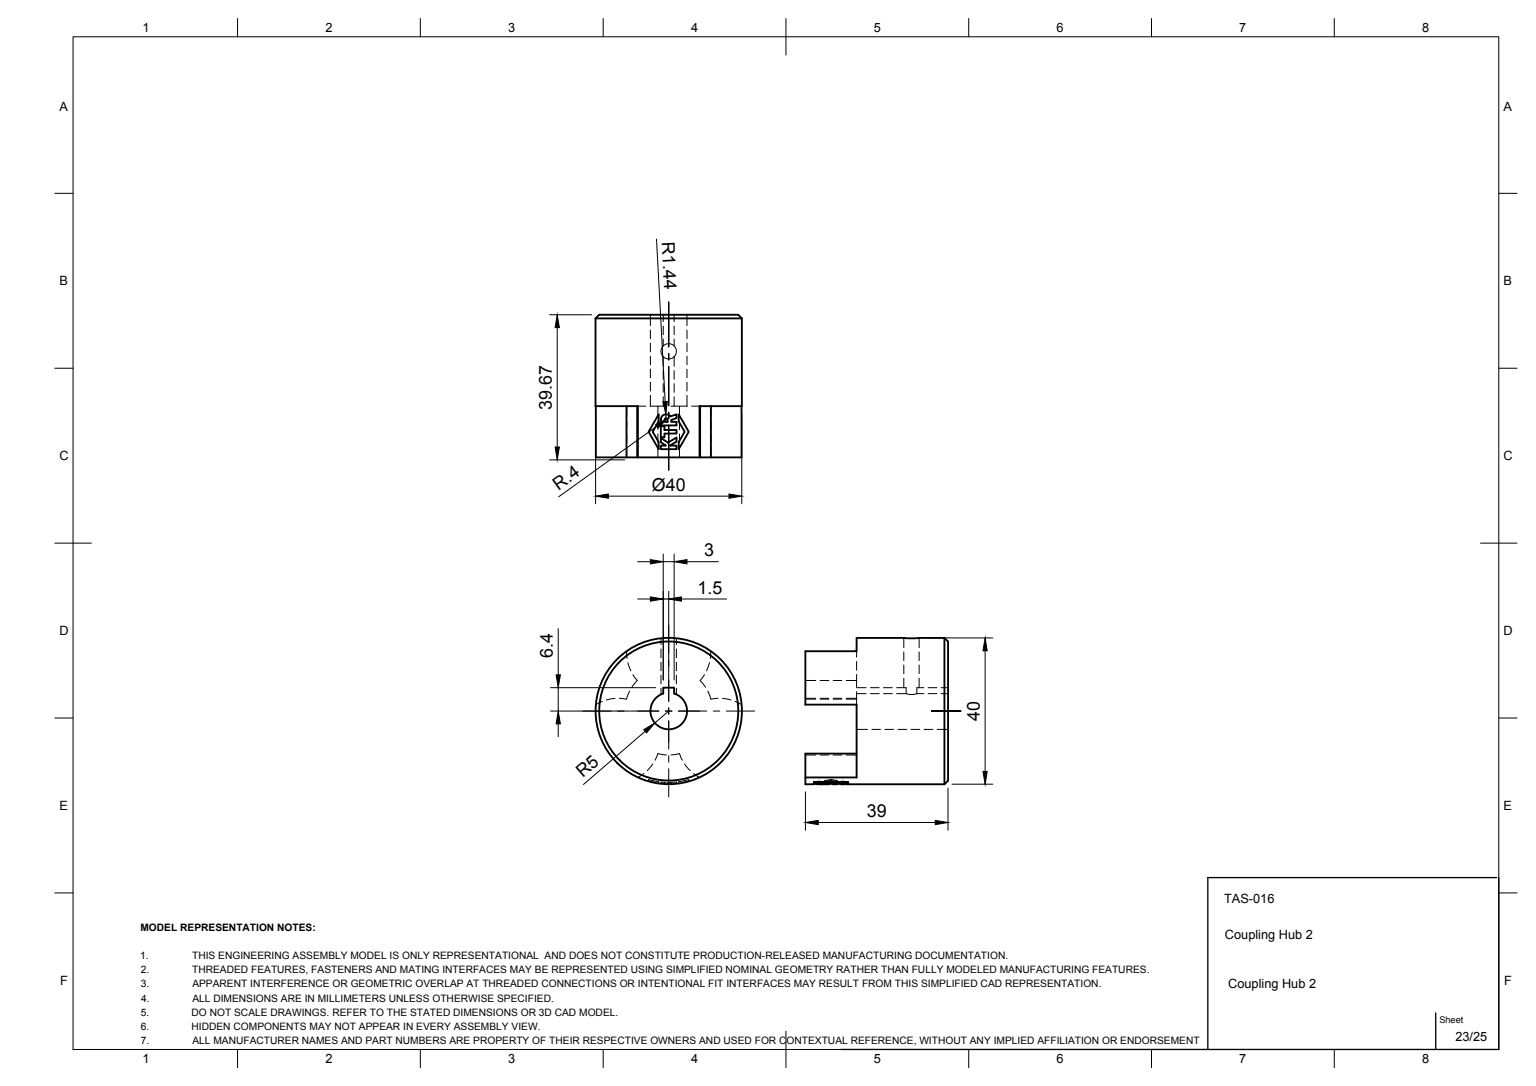
ISO-10303-21;
HEADER;
/* Generated by software containing ST-Developer
 * from STEP Tools, Inc. (www.steptools.com) 
 */

FILE_DESCRIPTION(
/* description */ ('STEP AP214'),
/* implementation_level */ '2;1');

FILE_NAME(
/* name */ 'Coupling Hub 2.step',
/* time_stamp */ '2026-11-15T14:55:55-08:00',
/* author */ (''),
/* organization */ (''),
/* preprocessor_version */ 'ST-DEVELOPER v20.2',
/* originating_system */ 'Autodesk Translation Framework v15.17.0.0',
/* authorisation */ '');

FILE_SCHEMA (('AUTOMOTIVE_DESIGN { 1 0 10303 214 3 1 1 }'));
ENDSEC;

DATA;
#10=MECHANICAL_DESIGN_GEOMETRIC_PRESENTATION_REPRESENTATION('',(#943),#57079);
#90=ELLIPSE('',#25887,40.0000000130718,20.0000000134373);
#91=ELLIPSE('',#25888,39.9999999264935,19.999999930827);
#92=ELLIPSE('',#25889,39.9999999974836,19.9999999977429);
#93=ELLIPSE('',#25890,40.0000000047116,20.0000000045204);
#94=ELLIPSE('',#25891,23.3867968076182,20.);
#95=ELLIPSE('',#25892,23.386796807644,20.);
#96=ELLIPSE('',#25896,24.1243589702644,20.);
#97=ELLIPSE('',#25897,24.124358970134,20.);
#98=ELLIPSE('',#25898,39.999999976902,19.9999999789991);
#99=ELLIPSE('',#25899,40.0000000049323,20.0000000047275);
#100=ELLIPSE('',#25900,39.9999999975502,19.999999997805);
#101=ELLIPSE('',#25901,39.9999999389236,19.9999999427079);
#102=ELLIPSE('',#25916,22.8021268874529,19.5);
#103=ELLIPSE('',#25919,22.8021268874277,19.5);
#104=ELLIPSE('',#25922,23.5212499960078,19.5);
#105=ELLIPSE('',#25932,23.5212499958807,19.5);
#106=ELLIPSE('',#25935,39.0000000024375,19.500000002367);
#107=ELLIPSE('',#25936,39.0000000667235,19.500000064201);
#108=ELLIPSE('',#25937,38.9999999995571,19.5000000004649);
#109=ELLIPSE('',#25938,38.999999996593,19.4999999968888);
#110=ELLIPSE('',#25947,38.9999999955418,19.4999999959037);
#111=ELLIPSE('',#25949,38.999999997527,19.4999999977637);
#112=ELLIPSE('',#25952,39.0000000253793,19.5000000249782);
#113=ELLIPSE('',#25954,39.0000000418424,19.5000000405918);
#851=B_SPLINE_CURVE_WITH_KNOTS('',3,(#52270,#52271,#52272,#52273,#52274,
#52275,#52276,#52277,#52278,#52279,#52280,#52281,#52282,#52283,#52284,#52285,
#52286,#52287),.UNSPECIFIED.,.F.,.F.,(4,2,2,2,2,2,2,2,4),(0.,0.0151925643701926,
0.0303851287403852,0.045584296496648,0.0607834642529108,0.0759910091953897,
0.0911985541378687,0.106391953286869,0.121585352435869),.UNSPECIFIED.);
#852=B_SPLINE_CURVE_WITH_KNOTS('',3,(#52369,#52370,#52371,#52372,#52373,
#52374,#52375,#52376,#52377,#52378,#52379),.UNSPECIFIED.,.F.,.F.,(4,2,3,
2,4),(-0.15830486583654,-0.080247501535826,0.,0.0802475015358259,0.15830486583654),
 .UNSPECIFIED.);
#853=B_SPLINE_CURVE_WITH_KNOTS('',3,(#52384,#52385,#52386,#52387,#52388,
#52389,#52390,#52391,#52392,#52393),.UNSPECIFIED.,.F.,.F.,(4,2,2,2,4),(0.483273505725753,
0.561330870026467,0.641578371562293,0.721825873098119,0.799883237398833),
 .UNSPECIFIED.);
#854=B_SPLINE_CURVE_WITH_KNOTS('',3,(#52421,#52422,#52423,#52424,#52425,
#52426,#52427,#52428,#52429,#52430,#52431,#52432,#52433,#52434,#52435,#52436,
#52437,#52438),.UNSPECIFIED.,.F.,.F.,(4,2,2,2,2,2,2,2,4),(0.316667444606564,
0.395834141831916,0.475000839057267,0.554167864135198,0.633334889213128,
0.712501914291059,0.791668939368989,0.870835636594341,0.950002333819692),
 .UNSPECIFIED.);
#855=B_SPLINE_CURVE_WITH_KNOTS('',3,(#52440,#52441,#52442,#52443,#52444,
#52445,#52446,#52447,#52448,#52449),.UNSPECIFIED.,.F.,.F.,(4,2,2,2,4),(-1.26666977842626,
-1.18750275334833,-1.10833572827039,-1.02916903104504,-0.950002333819692),
 .UNSPECIFIED.);
#856=B_SPLINE_CURVE_WITH_KNOTS('',3,(#52450,#52451,#52452,#52453,#52454,
#52455,#52456,#52457,#52458,#52459),.UNSPECIFIED.,.F.,.F.,(4,2,2,2,4),(0.950002333819692,
1.02916903104504,1.1083357282704,1.18750275334833,1.26666977842626),
 .UNSPECIFIED.);
#857=B_SPLINE_CURVE_WITH_KNOTS('',3,(#52465,#52466,#52467,#52468,#52469,
#52470,#52471,#52472,#52473,#52474,#52475,#52476,#52477,#52478,#52479,#52480),
 .UNSPECIFIED.,.F.,.F.,(4,2,2,2,2,2,2,4),(-0.779979052988675,-0.757912790448093,
-0.703814302563526,-0.64971581467896,-0.595510917659987,-0.541306020641014,
-0.487185868025911,-0.433065715410808),.UNSPECIFIED.);
#858=B_SPLINE_CURVE_WITH_KNOTS('',3,(#52703,#52704,#52705,#52706,#52707,
#52708,#52709,#52710,#52711,#52712,#52713,#52714,#52715,#52716,#52717,#52718),
 .UNSPECIFIED.,.F.,.F.,(4,2,2,2,2,2,2,4),(0.43308109743951,0.487202501340474,
0.541323905241438,0.595534461493003,0.649745017744569,0.703843614398011,
0.757942211051454,0.780009479202147),.UNSPECIFIED.);
#859=B_SPLINE_CURVE_WITH_KNOTS('',3,(#52750,#52751,#52752,#52753,#52754,
#52755,#52756,#52757,#52758,#52759,#52760,#52761,#52762,#52763,#52764,#52765,
#52766,#52767),.UNSPECIFIED.,.F.,.F.,(4,2,2,2,2,2,2,2,4),(0.121587491028333,
0.136780909575281,0.151974328122229,0.167182628159423,0.182390928196617,
0.197590414964019,0.212789901731421,0.227982441894043,0.243174982056666),
 .UNSPECIFIED.);
#883=SHAPE_REPRESENTATION_RELATIONSHIP('SRR','None',#57271,#912);
#912=ADVANCED_BREP_SHAPE_REPRESENTATION('',(#980),#57063);
#943=STYLED_ITEM('',(#57444),#980);
#980=MANIFOLD_SOLID_BREP('Body1',#24543);
#1149=FACE_BOUND('',#4239,.T.);
#1150=FACE_BOUND('',#4251,.T.);
#1151=FACE_BOUND('',#4264,.T.);
#1152=FACE_BOUND('',#4265,.T.);
#1153=FACE_BOUND('',#4266,.T.);
#1154=FACE_BOUND('',#4267,.T.);
#1155=FACE_BOUND('',#4268,.T.);
#1156=FACE_BOUND('',#4318,.T.);
#1609=PLANE('',#25821);
#1610=PLANE('',#25826);
#1611=PLANE('',#25833);
#1612=PLANE('',#25838);
#1613=PLANE('',#25855);
#1614=PLANE('',#25868);
#1615=PLANE('',#25869);
#1616=PLANE('',#25870);
#1617=PLANE('',#25872);
#1618=PLANE('',#25875);
#1619=PLANE('',#25876);
#1620=PLANE('',#25907);
#1621=PLANE('',#25908);
#1622=PLANE('',#25909);
#1623=PLANE('',#25910);
#1624=PLANE('',#25911);
#1625=PLANE('',#25912);
#1626=PLANE('',#25913);
#1627=PLANE('',#25914);
#1628=PLANE('',#25915);
#1629=PLANE('',#25917);
#1630=PLANE('',#25918);
#1631=PLANE('',#25920);
#1632=PLANE('',#25921);
#1633=PLANE('',#25923);
#1634=PLANE('',#25925);
#1635=PLANE('',#25926);
#1636=PLANE('',#25928);
#1637=PLANE('',#25929);
#1638=PLANE('',#25931);
#1639=PLANE('',#25939);
#1640=PLANE('',#25940);
#1641=PLANE('',#25941);
#1642=PLANE('',#25942);
#1643=PLANE('',#25943);
#1644=PLANE('',#25944);
#1645=PLANE('',#25945);
#1646=PLANE('',#25946);
#1647=PLANE('',#25948);
#1648=PLANE('',#25950);
#1649=PLANE('',#25951);
#1650=PLANE('',#25953);
#1651=PLANE('',#25956);
#1652=PLANE('',#25958);
#1653=PLANE('',#25959);
#1654=PLANE('',#25962);
#1655=PLANE('',#25963);
#1656=PLANE('',#25965);
#1657=PLANE('',#25966);
#1658=PLANE('',#25968);
#1659=PLANE('',#25969);
#1660=PLANE('',#25971);
#1661=PLANE('',#25973);
#2123=CONICAL_SURFACE('',#25829,19.5,0.785398163397448);
#2713=FACE_OUTER_BOUND('',#4237,.T.);
#2714=FACE_OUTER_BOUND('',#4238,.T.);
#2715=FACE_OUTER_BOUND('',#4240,.T.);
#2716=FACE_OUTER_BOUND('',#4241,.T.);
#2717=FACE_OUTER_BOUND('',#4242,.T.);
#2718=FACE_OUTER_BOUND('',#4243,.T.);
#2719=FACE_OUTER_BOUND('',#4244,.T.);
#2720=FACE_OUTER_BOUND('',#4245,.T.);
#2721=FACE_OUTER_BOUND('',#4246,.T.);
#2722=FACE_OUTER_BOUND('',#4247,.T.);
#2723=FACE_OUTER_BOUND('',#4248,.T.);
#2724=FACE_OUTER_BOUND('',#4249,.T.);
#2725=FACE_OUTER_BOUND('',#4250,.T.);
#2726=FACE_OUTER_BOUND('',#4252,.T.);
#2727=FACE_OUTER_BOUND('',#4253,.T.);
#2728=FACE_OUTER_BOUND('',#4254,.T.);
#2729=FACE_OUTER_BOUND('',#4255,.T.);
#2730=FACE_OUTER_BOUND('',#4256,.T.);
#2731=FACE_OUTER_BOUND('',#4257,.T.);
#2732=FACE_OUTER_BOUND('',#4258,.T.);
#2733=FACE_OUTER_BOUND('',#4259,.T.);
#2734=FACE_OUTER_BOUND('',#4260,.T.);
#2735=FACE_OUTER_BOUND('',#4261,.T.);
#2736=FACE_OUTER_BOUND('',#4262,.T.);
#2737=FACE_OUTER_BOUND('',#4263,.T.);
#2738=FACE_OUTER_BOUND('',#4269,.T.);
#2739=FACE_OUTER_BOUND('',#4270,.T.);
#2740=FACE_OUTER_BOUND('',#4271,.T.);
#2741=FACE_OUTER_BOUND('',#4272,.T.);
#2742=FACE_OUTER_BOUND('',#4273,.T.);
#2743=FACE_OUTER_BOUND('',#4274,.T.);
#2744=FACE_OUTER_BOUND('',#4275,.T.);
#2745=FACE_OUTER_BOUND('',#4276,.T.);
#2746=FACE_OUTER_BOUND('',#4277,.T.);
#2747=FACE_OUTER_BOUND('',#4278,.T.);
#2748=FACE_OUTER_BOUND('',#4279,.T.);
#2749=FACE_OUTER_BOUND('',#4280,.T.);
#2750=FACE_OUTER_BOUND('',#4281,.T.);
#2751=FACE_OUTER_BOUND('',#4282,.T.);
#2752=FACE_OUTER_BOUND('',#4283,.T.);
#2753=FACE_OUTER_BOUND('',#4284,.T.);
#2754=FACE_OUTER_BOUND('',#4285,.T.);
#2755=FACE_OUTER_BOUND('',#4286,.T.);
#2756=FACE_OUTER_BOUND('',#4287,.T.);
#2757=FACE_OUTER_BOUND('',#4288,.T.);
#2758=FACE_OUTER_BOUND('',#4289,.T.);
#2759=FACE_OUTER_BOUND('',#4290,.T.);
#2760=FACE_OUTER_BOUND('',#4291,.T.);
#2761=FACE_OUTER_BOUND('',#4292,.T.);
#2762=FACE_OUTER_BOUND('',#4293,.T.);
#2763=FACE_OUTER_BOUND('',#4294,.T.);
#2764=FACE_OUTER_BOUND('',#4295,.T.);
#2765=FACE_OUTER_BOUND('',#4296,.T.);
#2766=FACE_OUTER_BOUND('',#4297,.T.);
#2767=FACE_OUTER_BOUND('',#4298,.T.);
#2768=FACE_OUTER_BOUND('',#4299,.T.);
#2769=FACE_OUTER_BOUND('',#4300,.T.);
#2770=FACE_OUTER_BOUND('',#4301,.T.);
#2771=FACE_OUTER_BOUND('',#4302,.T.);
#2772=FACE_OUTER_BOUND('',#4303,.T.);
#2773=FACE_OUTER_BOUND('',#4304,.T.);
#2774=FACE_OUTER_BOUND('',#4305,.T.);
#2775=FACE_OUTER_BOUND('',#4306,.T.);
#2776=FACE_OUTER_BOUND('',#4307,.T.);
#2777=FACE_OUTER_BOUND('',#4308,.T.);
#2778=FACE_OUTER_BOUND('',#4309,.T.);
#2779=FACE_OUTER_BOUND('',#4310,.T.);
#2780=FACE_OUTER_BOUND('',#4311,.T.);
#2781=FACE_OUTER_BOUND('',#4312,.T.);
#2782=FACE_OUTER_BOUND('',#4313,.T.);
#2783=FACE_OUTER_BOUND('',#4314,.T.);
#2784=FACE_OUTER_BOUND('',#4315,.T.);
#2785=FACE_OUTER_BOUND('',#4316,.T.);
#2786=FACE_OUTER_BOUND('',#4317,.T.);
#4237=EDGE_LOOP('',(#18468,#18469,#18470,#18471));
#4238=EDGE_LOOP('',(#18472));
#4239=EDGE_LOOP('',(#18473,#18474,#18475,#18476));
#4240=EDGE_LOOP('',(#18477,#18478,#18479,#18480));
#4241=EDGE_LOOP('',(#18481,#18482,#18483,#18484));
#4242=EDGE_LOOP('',(#18485,#18486,#18487,#18488));
#4243=EDGE_LOOP('',(#18489,#18490,#18491,#18492));
#4244=EDGE_LOOP('',(#18493,#18494,#18495,#18496));
#4245=EDGE_LOOP('',(#18497,#18498,#18499,#18500));
#4246=EDGE_LOOP('',(#18501,#18502,#18503,#18504));
#4247=EDGE_LOOP('',(#18505,#18506,#18507,#18508));
#4248=EDGE_LOOP('',(#18509,#18510,#18511,#18512));
#4249=EDGE_LOOP('',(#18513,#18514,#18515,#18516));
#4250=EDGE_LOOP('',(#18517,#18518,#18519,#18520,#18521,#18522,#18523,#18524,
#18525,#18526,#18527,#18528,#18529));
#4251=EDGE_LOOP('',(#18530,#18531,#18532,#18533));
#4252=EDGE_LOOP('',(#18534,#18535,#18536,#18537));
#4253=EDGE_LOOP('',(#18538,#18539,#18540,#18541));
#4254=EDGE_LOOP('',(#18542,#18543,#18544,#18545));
#4255=EDGE_LOOP('',(#18546,#18547,#18548,#18549,#18550,#18551,#18552,#18553));
#4256=EDGE_LOOP('',(#18554,#18555,#18556,#18557));
#4257=EDGE_LOOP('',(#18558,#18559,#18560,#18561));
#4258=EDGE_LOOP('',(#18562,#18563,#18564,#18565));
#4259=EDGE_LOOP('',(#18566,#18567,#18568,#18569,#18570));
#4260=EDGE_LOOP('',(#18571,#18572,#18573,#18574));
#4261=EDGE_LOOP('',(#18575,#18576,#18577,#18578));
#4262=EDGE_LOOP('',(#18579,#18580,#18581,#18582,#18583,#18584,#18585,#18586,
#18587,#18588,#18589,#18590,#18591,#18592));
#4263=EDGE_LOOP('',(#18593,#18594,#18595,#18596,#18597,#18598,#18599,#18600,
#18601,#18602,#18603,#18604,#18605,#18606,#18607,#18608,#18609,#18610,#18611,
#18612,#18613));
#4264=EDGE_LOOP('',(#18614,#18615,#18616,#18617,#18618,#18619,#18620,#18621,
#18622));
#4265=EDGE_LOOP('',(#18623,#18624,#18625,#18626,#18627,#18628,#18629,#18630));
#4266=EDGE_LOOP('',(#18631,#18632,#18633,#18634,#18635,#18636));
#4267=EDGE_LOOP('',(#18637,#18638,#18639,#18640,#18641,#18642,#18643,#18644,
#18645,#18646,#18647));
#4268=EDGE_LOOP('',(#18648,#18649,#18650,#18651,#18652,#18653));
#4269=EDGE_LOOP('',(#18654,#18655,#18656,#18657,#18658,#18659,#18660,#18661));
#4270=EDGE_LOOP('',(#18662,#18663,#18664,#18665));
#4271=EDGE_LOOP('',(#18666,#18667,#18668,#18669));
#4272=EDGE_LOOP('',(#18670,#18671,#18672,#18673));
#4273=EDGE_LOOP('',(#18674,#18675,#18676,#18677));
#4274=EDGE_LOOP('',(#18678,#18679,#18680,#18681));
#4275=EDGE_LOOP('',(#18682,#18683,#18684,#18685));
#4276=EDGE_LOOP('',(#18686,#18687,#18688,#18689));
#4277=EDGE_LOOP('',(#18690,#18691,#18692,#18693));
#4278=EDGE_LOOP('',(#18694,#18695,#18696,#18697));
#4279=EDGE_LOOP('',(#18698,#18699,#18700,#18701));
#4280=EDGE_LOOP('',(#18702,#18703,#18704,#18705));
#4281=EDGE_LOOP('',(#18706,#18707,#18708,#18709));
#4282=EDGE_LOOP('',(#18710,#18711,#18712,#18713));
#4283=EDGE_LOOP('',(#18714,#18715,#18716,#18717));
#4284=EDGE_LOOP('',(#18718,#18719,#18720,#18721));
#4285=EDGE_LOOP('',(#18722,#18723,#18724,#18725));
#4286=EDGE_LOOP('',(#18726,#18727,#18728,#18729));
#4287=EDGE_LOOP('',(#18730,#18731,#18732,#18733));
#4288=EDGE_LOOP('',(#18734,#18735,#18736,#18737));
#4289=EDGE_LOOP('',(#18738,#18739,#18740,#18741,#18742,#18743,#18744,#18745,
#18746,#18747,#18748));
#4290=EDGE_LOOP('',(#18749,#18750,#18751,#18752,#18753,#18754));
#4291=EDGE_LOOP('',(#18755,#18756,#18757,#18758));
#4292=EDGE_LOOP('',(#18759,#18760,#18761,#18762));
#4293=EDGE_LOOP('',(#18763,#18764,#18765,#18766));
#4294=EDGE_LOOP('',(#18767,#18768,#18769,#18770));
#4295=EDGE_LOOP('',(#18771,#18772,#18773,#18774));
#4296=EDGE_LOOP('',(#18775,#18776,#18777,#18778));
#4297=EDGE_LOOP('',(#18779,#18780,#18781,#18782));
#4298=EDGE_LOOP('',(#18783,#18784,#18785,#18786));
#4299=EDGE_LOOP('',(#18787,#18788,#18789,#18790));
#4300=EDGE_LOOP('',(#18791,#18792,#18793,#18794));
#4301=EDGE_LOOP('',(#18795,#18796,#18797,#18798));
#4302=EDGE_LOOP('',(#18799,#18800,#18801,#18802));
#4303=EDGE_LOOP('',(#18803,#18804,#18805,#18806,#18807,#18808));
#4304=EDGE_LOOP('',(#18809,#18810,#18811,#18812));
#4305=EDGE_LOOP('',(#18813,#18814,#18815,#18816));
#4306=EDGE_LOOP('',(#18817,#18818,#18819,#18820));
#4307=EDGE_LOOP('',(#18821,#18822,#18823,#18824));
#4308=EDGE_LOOP('',(#18825,#18826,#18827,#18828));
#4309=EDGE_LOOP('',(#18829,#18830,#18831,#18832));
#4310=EDGE_LOOP('',(#18833,#18834,#18835,#18836));
#4311=EDGE_LOOP('',(#18837,#18838,#18839,#18840));
#4312=EDGE_LOOP('',(#18841,#18842,#18843,#18844));
#4313=EDGE_LOOP('',(#18845,#18846,#18847,#18848));
#4314=EDGE_LOOP('',(#18849,#18850,#18851,#18852));
#4315=EDGE_LOOP('',(#18853,#18854,#18855,#18856));
#4316=EDGE_LOOP('',(#18857,#18858,#18859,#18860));
#4317=EDGE_LOOP('',(#18861,#18862,#18863,#18864,#18865,#18866,#18867,#18868,
#18869));
#4318=EDGE_LOOP('',(#18870,#18871,#18872,#18873));
#5864=LINE('',#52255,#7831);
#5865=LINE('',#52257,#7832);
#5866=LINE('',#52259,#7833);
#5867=LINE('',#52264,#7834);
#5868=LINE('',#52268,#7835);
#5869=LINE('',#52289,#7836);
#5870=LINE('',#52313,#7837);
#5871=LINE('',#52314,#7838);
#5872=LINE('',#52317,#7839);
#5873=LINE('',#52320,#7840);
#5874=LINE('',#52323,#7841);
#5875=LINE('',#52326,#7842);
#5876=LINE('',#52329,#7843);
#5877=LINE('',#52333,#7844);
#5878=LINE('',#52338,#7845);
#5879=LINE('',#52353,#7846);
#5880=LINE('',#52357,#7847);
#5881=LINE('',#52358,#7848);
#5882=LINE('',#52360,#7849);
#5883=LINE('',#52362,#7850);
#5884=LINE('',#52364,#7851);
#5885=LINE('',#52367,#7852);
#5886=LINE('',#52380,#7853);
#5887=LINE('',#52382,#7854);
#5888=LINE('',#52394,#7855);
#5889=LINE('',#52397,#7856);
#5890=LINE('',#52398,#7857);
#5891=LINE('',#52401,#7858);
#5892=LINE('',#52402,#7859);
#5893=LINE('',#52406,#7860);
#5894=LINE('',#52411,#7861);
#5895=LINE('',#52414,#7862);
#5896=LINE('',#52416,#7863);
#5897=LINE('',#52419,#7864);
#5898=LINE('',#52461,#7865);
#5899=LINE('',#52462,#7866);
#5900=LINE('',#52484,#7867);
#5901=LINE('',#52488,#7868);
#5902=LINE('',#52492,#7869);
#5903=LINE('',#52495,#7870);
#5904=LINE('',#52500,#7871);
#5905=LINE('',#52504,#7872);
#5906=LINE('',#52508,#7873);
#5907=LINE('',#52511,#7874);
#5908=LINE('',#52514,#7875);
#5909=LINE('',#52520,#7876);
#5910=LINE('',#52528,#7877);
#5911=LINE('',#52534,#7878);
#5912=LINE('',#52538,#7879);
#5913=LINE('',#52544,#7880);
#5914=LINE('',#52550,#7881);
#5915=LINE('',#52556,#7882);
#5916=LINE('',#52563,#7883);
#5917=LINE('',#52567,#7884);
#5918=LINE('',#52571,#7885);
#5919=LINE('',#52574,#7886);
#5920=LINE('',#52576,#7887);
#5921=LINE('',#52577,#7888);
#5922=LINE('',#52579,#7889);
#5923=LINE('',#52581,#7890);
#5924=LINE('',#52583,#7891);
#5925=LINE('',#52585,#7892);
#5926=LINE('',#52587,#7893);
#5927=LINE('',#52589,#7894);
#5928=LINE('',#52593,#7895);
#5929=LINE('',#52596,#7896);
#5930=LINE('',#52599,#7897);
#5931=LINE('',#52600,#7898);
#5932=LINE('',#52603,#7899);
#5933=LINE('',#52607,#7900);
#5934=LINE('',#52609,#7901);
#5935=LINE('',#52610,#7902);
#5936=LINE('',#52613,#7903);
#5937=LINE('',#52617,#7904);
#5938=LINE('',#52621,#7905);
#5939=LINE('',#52622,#7906);
#5940=LINE('',#52625,#7907);
#5941=LINE('',#52629,#7908);
#5942=LINE('',#52630,#7909);
#5943=LINE('',#52641,#7910);
#5944=LINE('',#52647,#7911);
#5945=LINE('',#52650,#7912);
#5946=LINE('',#52651,#7913);
#5947=LINE('',#52653,#7914);
#5948=LINE('',#52655,#7915);
#5949=LINE('',#52657,#7916);
#5950=LINE('',#52659,#7917);
#5951=LINE('',#52663,#7918);
#5952=LINE('',#52665,#7919);
#5953=LINE('',#52666,#7920);
#5954=LINE('',#52669,#7921);
#5955=LINE('',#52673,#7922);
#5956=LINE('',#52677,#7923);
#5957=LINE('',#52678,#7924);
#5958=LINE('',#52682,#7925);
#5959=LINE('',#52688,#7926);
#5960=LINE('',#52691,#7927);
#5961=LINE('',#52694,#7928);
#5962=LINE('',#52695,#7929);
#5963=LINE('',#52698,#7930);
#5964=LINE('',#52702,#7931);
#5965=LINE('',#52721,#7932);
#5966=LINE('',#52722,#7933);
#5967=LINE('',#52725,#7934);
#5968=LINE('',#52728,#7935);
#5969=LINE('',#52731,#7936);
#5970=LINE('',#52732,#7937);
#5971=LINE('',#52735,#7938);
#5972=LINE('',#52739,#7939);
#5973=LINE('',#52740,#7940);
#5974=LINE('',#52743,#7941);
#5975=LINE('',#52746,#7942);
#5976=LINE('',#52749,#7943);
#5977=LINE('',#52769,#7944);
#7831=VECTOR('',#29980,1000.);
#7832=VECTOR('',#29981,1000.);
#7833=VECTOR('',#29982,1000.);
#7834=VECTOR('',#29989,19.5);
#7835=VECTOR('',#29992,1000.);
#7836=VECTOR('',#29993,1000.);
#7837=VECTOR('',#30020,1000.);
#7838=VECTOR('',#30021,1000.);
#7839=VECTOR('',#30024,1000.);
#7840=VECTOR('',#30027,1000.);
#7841=VECTOR('',#30030,1000.);
#7842=VECTOR('',#30033,1000.);
#7843=VECTOR('',#30036,1000.);
#7844=VECTOR('',#30041,1000.);
#7845=VECTOR('',#30048,1000.);
#7846=VECTOR('',#30065,1000.);
#7847=VECTOR('',#30068,1000.);
#7848=VECTOR('',#30069,1000.);
#7849=VECTOR('',#30072,1000.);
#7850=VECTOR('',#30075,1000.);
#7851=VECTOR('',#30078,1000.);
#7852=VECTOR('',#30081,1000.);
#7853=VECTOR('',#30082,1000.);
#7854=VECTOR('',#30083,1000.);
#7855=VECTOR('',#30084,1000.);
#7856=VECTOR('',#30087,1000.);
#7857=VECTOR('',#30088,1000.);
#7858=VECTOR('',#30091,1000.);
#7859=VECTOR('',#30092,1000.);
#7860=VECTOR('',#30097,1000.);
#7861=VECTOR('',#30102,1000.);
#7862=VECTOR('',#30107,1000.);
#7863=VECTOR('',#30110,1000.);
#7864=VECTOR('',#30113,2.1);
#7865=VECTOR('',#30116,20.);
#7866=VECTOR('',#30117,20.);
#7867=VECTOR('',#30120,1000.);
#7868=VECTOR('',#30123,1000.);
#7869=VECTOR('',#30126,1000.);
#7870=VECTOR('',#30129,1000.);
#7871=VECTOR('',#30132,1000.);
#7872=VECTOR('',#30135,1000.);
#7873=VECTOR('',#30138,1000.);
#7874=VECTOR('',#30141,1000.);
#7875=VECTOR('',#30142,1000.);
#7876=VECTOR('',#30147,1000.);
#7877=VECTOR('',#30154,1000.);
#7878=VECTOR('',#30159,1000.);
#7879=VECTOR('',#30162,1000.);
#7880=VECTOR('',#30167,1000.);
#7881=VECTOR('',#30172,1000.);
#7882=VECTOR('',#30177,1000.);
#7883=VECTOR('',#30184,1000.);
#7884=VECTOR('',#30187,1000.);
#7885=VECTOR('',#30190,1000.);
#7886=VECTOR('',#30193,1000.);
#7887=VECTOR('',#30196,1000.);
#7888=VECTOR('',#30197,1000.);
#7889=VECTOR('',#30200,1000.);
#7890=VECTOR('',#30203,1000.);
#7891=VECTOR('',#30206,1000.);
#7892=VECTOR('',#30209,1000.);
#7893=VECTOR('',#30212,1000.);
#7894=VECTOR('',#30215,1000.);
#7895=VECTOR('',#30220,1000.);
#7896=VECTOR('',#30223,1000.);
#7897=VECTOR('',#30226,1000.);
#7898=VECTOR('',#30227,1000.);
#7899=VECTOR('',#30230,1000.);
#7900=VECTOR('',#30235,1000.);
#7901=VECTOR('',#30236,1000.);
#7902=VECTOR('',#30237,1000.);
#7903=VECTOR('',#30240,1000.);
#7904=VECTOR('',#30245,1000.);
#7905=VECTOR('',#30250,1000.);
#7906=VECTOR('',#30251,1000.);
#7907=VECTOR('',#30254,1000.);
#7908=VECTOR('',#30259,1000.);
#7909=VECTOR('',#30260,1000.);
#7910=VECTOR('',#30275,1000.);
#7911=VECTOR('',#30280,1000.);
#7912=VECTOR('',#30285,1000.);
#7913=VECTOR('',#30286,1000.);
#7914=VECTOR('',#30289,1000.);
#7915=VECTOR('',#30292,1000.);
#7916=VECTOR('',#30295,1000.);
#7917=VECTOR('',#30298,1000.);
#7918=VECTOR('',#30303,1000.);
#7919=VECTOR('',#30304,1000.);
#7920=VECTOR('',#30305,1000.);
#7921=VECTOR('',#30308,1000.);
#7922=VECTOR('',#30313,1000.);
#7923=VECTOR('',#30318,1000.);
#7924=VECTOR('',#30319,1000.);
#7925=VECTOR('',#30324,1000.);
#7926=VECTOR('',#30333,1000.);
#7927=VECTOR('',#30336,1000.);
#7928=VECTOR('',#30339,1000.);
#7929=VECTOR('',#30340,1000.);
#7930=VECTOR('',#30343,1000.);
#7931=VECTOR('',#30348,1000.);
#7932=VECTOR('',#30351,1000.);
#7933=VECTOR('',#30352,1000.);
#7934=VECTOR('',#30355,1000.);
#7935=VECTOR('',#30358,1000.);
#7936=VECTOR('',#30361,1000.);
#7937=VECTOR('',#30362,1000.);
#7938=VECTOR('',#30365,1000.);
#7939=VECTOR('',#30370,1000.);
#7940=VECTOR('',#30371,1000.);
#7941=VECTOR('',#30374,1000.);
#7942=VECTOR('',#30379,1000.);
#7943=VECTOR('',#30382,1000.);
#7944=VECTOR('',#30385,1000.);
#9610=CIRCLE('',#25822,11.5);
#9611=CIRCLE('',#25823,20.);
#9612=CIRCLE('',#25824,11.5);
#9613=CIRCLE('',#25825,12.);
#9614=CIRCLE('',#25827,19.);
#9615=CIRCLE('',#25828,5.);
#9616=CIRCLE('',#25830,20.);
#9617=CIRCLE('',#25832,20.);
#9618=CIRCLE('',#25834,11.5);
#9619=CIRCLE('',#25835,20.);
#9620=CIRCLE('',#25836,11.5);
#9621=CIRCLE('',#25837,12.);
#9622=CIRCLE('',#25839,11.5);
#9623=CIRCLE('',#25840,12.);
#9624=CIRCLE('',#25841,11.5);
#9625=CIRCLE('',#25842,20.);
#9626=CIRCLE('',#25844,11.5);
#9627=CIRCLE('',#25846,12.);
#9628=CIRCLE('',#25848,12.);
#9629=CIRCLE('',#25850,12.);
#9630=CIRCLE('',#25852,11.5);
#9631=CIRCLE('',#25854,11.5);
#9632=CIRCLE('',#25856,20.);
#9633=CIRCLE('',#25857,11.5);
#9634=CIRCLE('',#25858,20.);
#9635=CIRCLE('',#25859,20.);
#9636=CIRCLE('',#25860,11.5);
#9637=CIRCLE('',#25861,20.);
#9638=CIRCLE('',#25862,11.5);
#9639=CIRCLE('',#25863,5.);
#9640=CIRCLE('',#25871,2.1);
#9641=CIRCLE('',#25873,2.1);
#9642=CIRCLE('',#25874,2.1);
#9643=CIRCLE('',#25879,22.3311974134124);
#9644=CIRCLE('',#25880,22.32884051476);
#9645=CIRCLE('',#25881,20.);
#9646=CIRCLE('',#25882,20.);
#9647=CIRCLE('',#25883,20.);
#9648=CIRCLE('',#25884,20.);
#9649=CIRCLE('',#25885,20.);
#9650=CIRCLE('',#25886,20.);
#9651=CIRCLE('',#25893,20.);
#9652=CIRCLE('',#25894,20.);
#9653=CIRCLE('',#25895,20.);
#9654=CIRCLE('',#25903,19.5);
#9655=CIRCLE('',#25904,19.5);
#9656=CIRCLE('',#25905,19.5);
#9657=CIRCLE('',#25906,19.5);
#9658=CIRCLE('',#25924,19.5);
#9659=CIRCLE('',#25927,19.5);
#9660=CIRCLE('',#25930,19.5);
#9661=CIRCLE('',#25957,21.7696935948967);
#9662=CIRCLE('',#25960,21.7721107487055);
#9663=CIRCLE('',#25964,19.5);
#9664=CIRCLE('',#25967,19.5);
#9665=CIRCLE('',#25970,19.5);
#11088=VERTEX_POINT('',#52242);
#11089=VERTEX_POINT('',#52243);
#11090=VERTEX_POINT('',#52245);
#11091=VERTEX_POINT('',#52247);
#11092=VERTEX_POINT('',#52251);
#11093=VERTEX_POINT('',#52253);
#11094=VERTEX_POINT('',#52254);
#11095=VERTEX_POINT('',#52256);
#11096=VERTEX_POINT('',#52258);
#11097=VERTEX_POINT('',#52262);
#11098=VERTEX_POINT('',#52266);
#11099=VERTEX_POINT('',#52267);
#11100=VERTEX_POINT('',#52269);
#11101=VERTEX_POINT('',#52288);
#11102=VERTEX_POINT('',#52292);
#11103=VERTEX_POINT('',#52293);
#11104=VERTEX_POINT('',#52295);
#11105=VERTEX_POINT('',#52297);
#11106=VERTEX_POINT('',#52301);
#11107=VERTEX_POINT('',#52302);
#11108=VERTEX_POINT('',#52304);
#11109=VERTEX_POINT('',#52306);
#11110=VERTEX_POINT('',#52310);
#11111=VERTEX_POINT('',#52311);
#11112=VERTEX_POINT('',#52316);
#11113=VERTEX_POINT('',#52318);
#11114=VERTEX_POINT('',#52322);
#11115=VERTEX_POINT('',#52324);
#11116=VERTEX_POINT('',#52328);
#11117=VERTEX_POINT('',#52332);
#11118=VERTEX_POINT('',#52336);
#11119=VERTEX_POINT('',#52340);
#11120=VERTEX_POINT('',#52342);
#11121=VERTEX_POINT('',#52344);
#11122=VERTEX_POINT('',#52346);
#11123=VERTEX_POINT('',#52351);
#11124=VERTEX_POINT('',#52352);
#11125=VERTEX_POINT('',#52354);
#11126=VERTEX_POINT('',#52356);
#11127=VERTEX_POINT('',#52366);
#11128=VERTEX_POINT('',#52368);
#11129=VERTEX_POINT('',#52381);
#11130=VERTEX_POINT('',#52383);
#11131=VERTEX_POINT('',#52396);
#11132=VERTEX_POINT('',#52400);
#11133=VERTEX_POINT('',#52404);
#11134=VERTEX_POINT('',#52408);
#11135=VERTEX_POINT('',#52410);
#11136=VERTEX_POINT('',#52418);
#11137=VERTEX_POINT('',#52420);
#11138=VERTEX_POINT('',#52439);
#11139=VERTEX_POINT('',#52463);
#11140=VERTEX_POINT('',#52464);
#11141=VERTEX_POINT('',#52481);
#11142=VERTEX_POINT('',#52483);
#11143=VERTEX_POINT('',#52485);
#11144=VERTEX_POINT('',#52487);
#11145=VERTEX_POINT('',#52489);
#11146=VERTEX_POINT('',#52491);
#11147=VERTEX_POINT('',#52493);
#11148=VERTEX_POINT('',#52496);
#11149=VERTEX_POINT('',#52497);
#11150=VERTEX_POINT('',#52499);
#11151=VERTEX_POINT('',#52501);
#11152=VERTEX_POINT('',#52503);
#11153=VERTEX_POINT('',#52505);
#11154=VERTEX_POINT('',#52507);
#11155=VERTEX_POINT('',#52509);
#11156=VERTEX_POINT('',#52512);
#11157=VERTEX_POINT('',#52513);
#11158=VERTEX_POINT('',#52515);
#11159=VERTEX_POINT('',#52517);
#11160=VERTEX_POINT('',#52519);
#11161=VERTEX_POINT('',#52521);
#11162=VERTEX_POINT('',#52524);
#11163=VERTEX_POINT('',#52525);
#11164=VERTEX_POINT('',#52527);
#11165=VERTEX_POINT('',#52529);
#11166=VERTEX_POINT('',#52531);
#11167=VERTEX_POINT('',#52533);
#11168=VERTEX_POINT('',#52535);
#11169=VERTEX_POINT('',#52537);
#11170=VERTEX_POINT('',#52539);
#11171=VERTEX_POINT('',#52541);
#11172=VERTEX_POINT('',#52543);
#11173=VERTEX_POINT('',#52546);
#11174=VERTEX_POINT('',#52547);
#11175=VERTEX_POINT('',#52549);
#11176=VERTEX_POINT('',#52551);
#11177=VERTEX_POINT('',#52553);
#11178=VERTEX_POINT('',#52555);
#11179=VERTEX_POINT('',#52559);
#11180=VERTEX_POINT('',#52560);
#11181=VERTEX_POINT('',#52562);
#11182=VERTEX_POINT('',#52564);
#11183=VERTEX_POINT('',#52566);
#11184=VERTEX_POINT('',#52568);
#11185=VERTEX_POINT('',#52570);
#11186=VERTEX_POINT('',#52572);
#11187=VERTEX_POINT('',#52592);
#11188=VERTEX_POINT('',#52594);
#11189=VERTEX_POINT('',#52598);
#11190=VERTEX_POINT('',#52602);
#11191=VERTEX_POINT('',#52606);
#11192=VERTEX_POINT('',#52608);
#11193=VERTEX_POINT('',#52612);
#11194=VERTEX_POINT('',#52616);
#11195=VERTEX_POINT('',#52620);
#11196=VERTEX_POINT('',#52624);
#11197=VERTEX_POINT('',#52628);
#11198=VERTEX_POINT('',#52637);
#11199=VERTEX_POINT('',#52638);
#11200=VERTEX_POINT('',#52640);
#11201=VERTEX_POINT('',#52642);
#11202=VERTEX_POINT('',#52644);
#11203=VERTEX_POINT('',#52646);
#11204=VERTEX_POINT('',#52662);
#11205=VERTEX_POINT('',#52664);
#11206=VERTEX_POINT('',#52668);
#11207=VERTEX_POINT('',#52672);
#11208=VERTEX_POINT('',#52676);
#11209=VERTEX_POINT('',#52680);
#11210=VERTEX_POINT('',#52687);
#11211=VERTEX_POINT('',#52689);
#11212=VERTEX_POINT('',#52693);
#11213=VERTEX_POINT('',#52697);
#11214=VERTEX_POINT('',#52701);
#11215=VERTEX_POINT('',#52720);
#11216=VERTEX_POINT('',#52724);
#11217=VERTEX_POINT('',#52726);
#11218=VERTEX_POINT('',#52730);
#11219=VERTEX_POINT('',#52734);
#11220=VERTEX_POINT('',#52738);
#11221=VERTEX_POINT('',#52742);
#11222=VERTEX_POINT('',#52748);
#13779=EDGE_CURVE('',#11088,#11089,#9610,.T.);
#13780=EDGE_CURVE('',#11090,#11089,#9611,.T.);
#13781=EDGE_CURVE('',#11090,#11091,#9612,.T.);
#13782=EDGE_CURVE('',#11091,#11088,#9613,.T.);
#13783=EDGE_CURVE('',#11092,#11092,#9614,.T.);
#13784=EDGE_CURVE('',#11093,#11094,#5864,.T.);
#13785=EDGE_CURVE('',#11094,#11095,#5865,.T.);
#13786=EDGE_CURVE('',#11095,#11096,#5866,.T.);
#13787=EDGE_CURVE('',#11096,#11093,#9615,.T.);
#13788=EDGE_CURVE('',#11097,#11097,#9616,.T.);
#13789=EDGE_CURVE('',#11097,#11092,#5867,.T.);
#13790=EDGE_CURVE('',#11098,#11099,#5868,.T.);
#13791=EDGE_CURVE('',#11099,#11100,#851,.T.);
#13792=EDGE_CURVE('',#11100,#11101,#5869,.T.);
#13793=EDGE_CURVE('',#11101,#11098,#9617,.T.);
#13794=EDGE_CURVE('',#11102,#11103,#9618,.T.);
#13795=EDGE_CURVE('',#11104,#11103,#9619,.T.);
#13796=EDGE_CURVE('',#11104,#11105,#9620,.T.);
#13797=EDGE_CURVE('',#11105,#11102,#9621,.T.);
#13798=EDGE_CURVE('',#11106,#11107,#9622,.T.);
#13799=EDGE_CURVE('',#11107,#11108,#9623,.T.);
#13800=EDGE_CURVE('',#11108,#11109,#9624,.T.);
#13801=EDGE_CURVE('',#11106,#11109,#9625,.T.);
#13802=EDGE_CURVE('',#11110,#11111,#9626,.T.);
#13803=EDGE_CURVE('',#11089,#11111,#5870,.T.);
#13804=EDGE_CURVE('',#11110,#11088,#5871,.T.);
#13805=EDGE_CURVE('',#11107,#11112,#5872,.T.);
#13806=EDGE_CURVE('',#11112,#11113,#9627,.T.);
#13807=EDGE_CURVE('',#11113,#11108,#5873,.T.);
#13808=EDGE_CURVE('',#11105,#11114,#5874,.T.);
#13809=EDGE_CURVE('',#11114,#11115,#9628,.T.);
#13810=EDGE_CURVE('',#11115,#11102,#5875,.T.);
#13811=EDGE_CURVE('',#11091,#11116,#5876,.T.);
#13812=EDGE_CURVE('',#11116,#11110,#9629,.T.);
#13813=EDGE_CURVE('',#11117,#11104,#5877,.T.);
#13814=EDGE_CURVE('',#11117,#11114,#9630,.T.);
#13815=EDGE_CURVE('',#11113,#11118,#9631,.T.);
#13816=EDGE_CURVE('',#11109,#11118,#5878,.T.);
#13817=EDGE_CURVE('',#11111,#11119,#9632,.T.);
#13818=EDGE_CURVE('',#11120,#11116,#9633,.T.);
#13819=EDGE_CURVE('',#11121,#11120,#9634,.T.);
#13820=EDGE_CURVE('',#11122,#11121,#9635,.T.);
#13821=EDGE_CURVE('',#11115,#11122,#9636,.T.);
#13822=EDGE_CURVE('',#11118,#11117,#9637,.T.);
#13823=EDGE_CURVE('',#11119,#11112,#9638,.T.);
#13824=EDGE_CURVE('',#11123,#11124,#5879,.T.);
#13825=EDGE_CURVE('',#11124,#11125,#9639,.T.);
#13826=EDGE_CURVE('',#11125,#11126,#5880,.T.);
#13827=EDGE_CURVE('',#11126,#11123,#5881,.T.);
#13828=EDGE_CURVE('',#11120,#11090,#5882,.T.);
#13829=EDGE_CURVE('',#11103,#11122,#5883,.T.);
#13830=EDGE_CURVE('',#11119,#11106,#5884,.T.);
#13831=EDGE_CURVE('',#11127,#11124,#5885,.T.);
#13832=EDGE_CURVE('',#11128,#11127,#852,.T.);
#13833=EDGE_CURVE('',#11093,#11128,#5886,.T.);
#13834=EDGE_CURVE('',#11129,#11096,#5887,.T.);
#13835=EDGE_CURVE('',#11130,#11129,#853,.T.);
#13836=EDGE_CURVE('',#11125,#11130,#5888,.T.);
#13837=EDGE_CURVE('',#11131,#11130,#5889,.T.);
#13838=EDGE_CURVE('',#11131,#11126,#5890,.T.);
#13839=EDGE_CURVE('',#11129,#11132,#5891,.T.);
#13840=EDGE_CURVE('',#11095,#11132,#5892,.T.);
#13841=EDGE_CURVE('',#11133,#11131,#9640,.T.);
#13842=EDGE_CURVE('',#11123,#11133,#5893,.T.);
#13843=EDGE_CURVE('',#11132,#11134,#9641,.T.);
#13844=EDGE_CURVE('',#11135,#11094,#5894,.T.);
#13845=EDGE_CURVE('',#11134,#11135,#9642,.T.);
#13846=EDGE_CURVE('',#11127,#11133,#5895,.T.);
#13847=EDGE_CURVE('',#11135,#11128,#5896,.T.);
#13848=EDGE_CURVE('',#11134,#11136,#5897,.T.);
#13849=EDGE_CURVE('',#11137,#11136,#854,.T.);
#13850=EDGE_CURVE('',#11138,#11137,#855,.T.);
#13851=EDGE_CURVE('',#11136,#11138,#856,.T.);
#13852=EDGE_CURVE('',#11097,#11136,#5898,.T.);
#13853=EDGE_CURVE('',#11137,#11121,#5899,.T.);
#13854=EDGE_CURVE('',#11139,#11140,#857,.F.);
#13855=EDGE_CURVE('',#11140,#11141,#9643,.T.);
#13856=EDGE_CURVE('',#11141,#11142,#5900,.T.);
#13857=EDGE_CURVE('',#11142,#11143,#9644,.T.);
#13858=EDGE_CURVE('',#11143,#11144,#5901,.T.);
#13859=EDGE_CURVE('',#11144,#11145,#9645,.T.);
#13860=EDGE_CURVE('',#11145,#11146,#5902,.T.);
#13861=EDGE_CURVE('',#11146,#11147,#9646,.T.);
#13862=EDGE_CURVE('',#11147,#11139,#5903,.T.);
#13863=EDGE_CURVE('',#11148,#11149,#9647,.T.);
#13864=EDGE_CURVE('',#11149,#11150,#5904,.T.);
#13865=EDGE_CURVE('',#11150,#11151,#9648,.T.);
#13866=EDGE_CURVE('',#11151,#11152,#5905,.T.);
#13867=EDGE_CURVE('',#11152,#11153,#9649,.T.);
#13868=EDGE_CURVE('',#11153,#11154,#5906,.T.);
#13869=EDGE_CURVE('',#11154,#11155,#9650,.T.);
#13870=EDGE_CURVE('',#11155,#11148,#5907,.T.);
#13871=EDGE_CURVE('',#11156,#11157,#5908,.T.);
#13872=EDGE_CURVE('',#11157,#11158,#90,.T.);
#13873=EDGE_CURVE('',#11158,#11159,#91,.T.);
#13874=EDGE_CURVE('',#11159,#11160,#5909,.T.);
#13875=EDGE_CURVE('',#11160,#11161,#92,.T.);
#13876=EDGE_CURVE('',#11161,#11156,#93,.T.);
#13877=EDGE_CURVE('',#11162,#11163,#94,.F.);
#13878=EDGE_CURVE('',#11163,#11164,#5910,.T.);
#13879=EDGE_CURVE('',#11164,#11165,#95,.T.);
#13880=EDGE_CURVE('',#11165,#11166,#9651,.T.);
#13881=EDGE_CURVE('',#11166,#11167,#5911,.T.);
#13882=EDGE_CURVE('',#11167,#11168,#9652,.T.);
#13883=EDGE_CURVE('',#11168,#11169,#5912,.T.);
#13884=EDGE_CURVE('',#11169,#11170,#9653,.T.);
#13885=EDGE_CURVE('',#11170,#11171,#96,.T.);
#13886=EDGE_CURVE('',#11171,#11172,#5913,.T.);
#13887=EDGE_CURVE('',#11172,#11162,#97,.T.);
#13888=EDGE_CURVE('',#11173,#11174,#98,.T.);
#13889=EDGE_CURVE('',#11174,#11175,#5914,.T.);
#13890=EDGE_CURVE('',#11175,#11176,#99,.T.);
#13891=EDGE_CURVE('',#11176,#11177,#100,.T.);
#13892=EDGE_CURVE('',#11177,#11178,#5915,.T.);
#13893=EDGE_CURVE('',#11178,#11173,#101,.T.);
#13894=EDGE_CURVE('',#11179,#11180,#9654,.T.);
#13895=EDGE_CURVE('',#11180,#11181,#5916,.T.);
#13896=EDGE_CURVE('',#11181,#11182,#9655,.T.);
#13897=EDGE_CURVE('',#11182,#11183,#5917,.T.);
#13898=EDGE_CURVE('',#11183,#11184,#9656,.T.);
#13899=EDGE_CURVE('',#11184,#11185,#5918,.T.);
#13900=EDGE_CURVE('',#11185,#11186,#9657,.T.);
#13901=EDGE_CURVE('',#11186,#11179,#5919,.T.);
#13902=EDGE_CURVE('',#11186,#11150,#5920,.T.);
#13903=EDGE_CURVE('',#11185,#11151,#5921,.T.);
#13904=EDGE_CURVE('',#11179,#11149,#5922,.T.);
#13905=EDGE_CURVE('',#11184,#11152,#5923,.T.);
#13906=EDGE_CURVE('',#11183,#11153,#5924,.T.);
#13907=EDGE_CURVE('',#11182,#11154,#5925,.T.);
#13908=EDGE_CURVE('',#11181,#11155,#5926,.T.);
#13909=EDGE_CURVE('',#11180,#11148,#5927,.T.);
#13910=EDGE_CURVE('',#11187,#11164,#5928,.T.);
#13911=EDGE_CURVE('',#11188,#11187,#102,.T.);
#13912=EDGE_CURVE('',#11188,#11165,#5929,.T.);
#13913=EDGE_CURVE('',#11189,#11163,#5930,.T.);
#13914=EDGE_CURVE('',#11187,#11189,#5931,.T.);
#13915=EDGE_CURVE('',#11190,#11162,#5932,.T.);
#13916=EDGE_CURVE('',#11189,#11190,#103,.F.);
#13917=EDGE_CURVE('',#11191,#11171,#5933,.T.);
#13918=EDGE_CURVE('',#11192,#11191,#5934,.T.);
#13919=EDGE_CURVE('',#11192,#11172,#5935,.T.);
#13920=EDGE_CURVE('',#11193,#11170,#5936,.T.);
#13921=EDGE_CURVE('',#11191,#11193,#104,.T.);
#13922=EDGE_CURVE('',#11194,#11169,#5937,.T.);
#13923=EDGE_CURVE('',#11193,#11194,#9658,.T.);
#13924=EDGE_CURVE('',#11195,#11168,#5938,.T.);
#13925=EDGE_CURVE('',#11194,#11195,#5939,.T.);
#13926=EDGE_CURVE('',#11196,#11167,#5940,.T.);
#13927=EDGE_CURVE('',#11195,#11196,#9659,.T.);
#13928=EDGE_CURVE('',#11197,#11166,#5941,.T.);
#13929=EDGE_CURVE('',#11196,#11197,#5942,.T.);
#13930=EDGE_CURVE('',#11197,#11188,#9660,.T.);
#13931=EDGE_CURVE('',#11190,#11192,#105,.T.);
#13932=EDGE_CURVE('',#11198,#11199,#106,.T.);
#13933=EDGE_CURVE('',#11199,#11200,#5943,.T.);
#13934=EDGE_CURVE('',#11200,#11201,#107,.T.);
#13935=EDGE_CURVE('',#11201,#11202,#108,.T.);
#13936=EDGE_CURVE('',#11202,#11203,#5944,.T.);
#13937=EDGE_CURVE('',#11203,#11198,#109,.T.);
#13938=EDGE_CURVE('',#11201,#11158,#5945,.T.);
#13939=EDGE_CURVE('',#11200,#11159,#5946,.T.);
#13940=EDGE_CURVE('',#11202,#11157,#5947,.T.);
#13941=EDGE_CURVE('',#11199,#11160,#5948,.T.);
#13942=EDGE_CURVE('',#11198,#11161,#5949,.T.);
#13943=EDGE_CURVE('',#11203,#11156,#5950,.T.);
#13944=EDGE_CURVE('',#11204,#11177,#5951,.T.);
#13945=EDGE_CURVE('',#11205,#11204,#5952,.T.);
#13946=EDGE_CURVE('',#11205,#11178,#5953,.T.);
#13947=EDGE_CURVE('',#11206,#11176,#5954,.T.);
#13948=EDGE_CURVE('',#11204,#11206,#110,.T.);
#13949=EDGE_CURVE('',#11207,#11175,#5955,.T.);
#13950=EDGE_CURVE('',#11206,#11207,#111,.T.);
#13951=EDGE_CURVE('',#11208,#11174,#5956,.T.);
#13952=EDGE_CURVE('',#11207,#11208,#5957,.T.);
#13953=EDGE_CURVE('',#11209,#11205,#112,.T.);
#13954=EDGE_CURVE('',#11209,#11173,#5958,.T.);
#13955=EDGE_CURVE('',#11208,#11209,#113,.T.);
#13956=EDGE_CURVE('',#11210,#11142,#5959,.T.);
#13957=EDGE_CURVE('',#11211,#11210,#9661,.T.);
#13958=EDGE_CURVE('',#11211,#11143,#5960,.T.);
#13959=EDGE_CURVE('',#11212,#11141,#5961,.T.);
#13960=EDGE_CURVE('',#11210,#11212,#5962,.T.);
#13961=EDGE_CURVE('',#11213,#11140,#5963,.T.);
#13962=EDGE_CURVE('',#11212,#11213,#9662,.T.);
#13963=EDGE_CURVE('',#11214,#11139,#5964,.T.);
#13964=EDGE_CURVE('',#11213,#11214,#858,.F.);
#13965=EDGE_CURVE('',#11215,#11147,#5965,.T.);
#13966=EDGE_CURVE('',#11214,#11215,#5966,.T.);
#13967=EDGE_CURVE('',#11216,#11101,#5967,.T.);
#13968=EDGE_CURVE('',#11217,#11216,#9663,.T.);
#13969=EDGE_CURVE('',#11217,#11098,#5968,.T.);
#13970=EDGE_CURVE('',#11218,#11100,#5969,.T.);
#13971=EDGE_CURVE('',#11216,#11218,#5970,.T.);
#13972=EDGE_CURVE('',#11219,#11146,#5971,.T.);
#13973=EDGE_CURVE('',#11215,#11219,#9664,.T.);
#13974=EDGE_CURVE('',#11220,#11145,#5972,.T.);
#13975=EDGE_CURVE('',#11219,#11220,#5973,.T.);
#13976=EDGE_CURVE('',#11221,#11144,#5974,.T.);
#13977=EDGE_CURVE('',#11220,#11221,#9665,.T.);
#13978=EDGE_CURVE('',#11221,#11211,#5975,.T.);
#13979=EDGE_CURVE('',#11222,#11099,#5976,.T.);
#13980=EDGE_CURVE('',#11218,#11222,#859,.T.);
#13981=EDGE_CURVE('',#11222,#11217,#5977,.T.);
#18468=ORIENTED_EDGE('',*,*,#13779,.T.);
#18469=ORIENTED_EDGE('',*,*,#13780,.F.);
#18470=ORIENTED_EDGE('',*,*,#13781,.T.);
#18471=ORIENTED_EDGE('',*,*,#13782,.T.);
#18472=ORIENTED_EDGE('',*,*,#13783,.T.);
#18473=ORIENTED_EDGE('',*,*,#13784,.T.);
#18474=ORIENTED_EDGE('',*,*,#13785,.T.);
#18475=ORIENTED_EDGE('',*,*,#13786,.T.);
#18476=ORIENTED_EDGE('',*,*,#13787,.T.);
#18477=ORIENTED_EDGE('',*,*,#13788,.T.);
#18478=ORIENTED_EDGE('',*,*,#13789,.T.);
#18479=ORIENTED_EDGE('',*,*,#13783,.F.);
#18480=ORIENTED_EDGE('',*,*,#13789,.F.);
#18481=ORIENTED_EDGE('',*,*,#13790,.T.);
#18482=ORIENTED_EDGE('',*,*,#13791,.T.);
#18483=ORIENTED_EDGE('',*,*,#13792,.T.);
#18484=ORIENTED_EDGE('',*,*,#13793,.T.);
#18485=ORIENTED_EDGE('',*,*,#13794,.T.);
#18486=ORIENTED_EDGE('',*,*,#13795,.F.);
#18487=ORIENTED_EDGE('',*,*,#13796,.T.);
#18488=ORIENTED_EDGE('',*,*,#13797,.T.);
#18489=ORIENTED_EDGE('',*,*,#13798,.T.);
#18490=ORIENTED_EDGE('',*,*,#13799,.T.);
#18491=ORIENTED_EDGE('',*,*,#13800,.T.);
#18492=ORIENTED_EDGE('',*,*,#13801,.F.);
#18493=ORIENTED_EDGE('',*,*,#13802,.T.);
#18494=ORIENTED_EDGE('',*,*,#13803,.F.);
#18495=ORIENTED_EDGE('',*,*,#13779,.F.);
#18496=ORIENTED_EDGE('',*,*,#13804,.F.);
#18497=ORIENTED_EDGE('',*,*,#13799,.F.);
#18498=ORIENTED_EDGE('',*,*,#13805,.T.);
#18499=ORIENTED_EDGE('',*,*,#13806,.T.);
#18500=ORIENTED_EDGE('',*,*,#13807,.T.);
#18501=ORIENTED_EDGE('',*,*,#13808,.T.);
#18502=ORIENTED_EDGE('',*,*,#13809,.T.);
#18503=ORIENTED_EDGE('',*,*,#13810,.T.);
#18504=ORIENTED_EDGE('',*,*,#13797,.F.);
#18505=ORIENTED_EDGE('',*,*,#13804,.T.);
#18506=ORIENTED_EDGE('',*,*,#13782,.F.);
#18507=ORIENTED_EDGE('',*,*,#13811,.T.);
#18508=ORIENTED_EDGE('',*,*,#13812,.T.);
#18509=ORIENTED_EDGE('',*,*,#13796,.F.);
#18510=ORIENTED_EDGE('',*,*,#13813,.F.);
#18511=ORIENTED_EDGE('',*,*,#13814,.T.);
#18512=ORIENTED_EDGE('',*,*,#13808,.F.);
#18513=ORIENTED_EDGE('',*,*,#13815,.T.);
#18514=ORIENTED_EDGE('',*,*,#13816,.F.);
#18515=ORIENTED_EDGE('',*,*,#13800,.F.);
#18516=ORIENTED_EDGE('',*,*,#13807,.F.);
#18517=ORIENTED_EDGE('',*,*,#13817,.F.);
#18518=ORIENTED_EDGE('',*,*,#13802,.F.);
#18519=ORIENTED_EDGE('',*,*,#13812,.F.);
#18520=ORIENTED_EDGE('',*,*,#13818,.F.);
#18521=ORIENTED_EDGE('',*,*,#13819,.F.);
#18522=ORIENTED_EDGE('',*,*,#13820,.F.);
#18523=ORIENTED_EDGE('',*,*,#13821,.F.);
#18524=ORIENTED_EDGE('',*,*,#13809,.F.);
#18525=ORIENTED_EDGE('',*,*,#13814,.F.);
#18526=ORIENTED_EDGE('',*,*,#13822,.F.);
#18527=ORIENTED_EDGE('',*,*,#13815,.F.);
#18528=ORIENTED_EDGE('',*,*,#13806,.F.);
#18529=ORIENTED_EDGE('',*,*,#13823,.F.);
#18530=ORIENTED_EDGE('',*,*,#13824,.T.);
#18531=ORIENTED_EDGE('',*,*,#13825,.T.);
#18532=ORIENTED_EDGE('',*,*,#13826,.T.);
#18533=ORIENTED_EDGE('',*,*,#13827,.T.);
#18534=ORIENTED_EDGE('',*,*,#13781,.F.);
#18535=ORIENTED_EDGE('',*,*,#13828,.F.);
#18536=ORIENTED_EDGE('',*,*,#13818,.T.);
#18537=ORIENTED_EDGE('',*,*,#13811,.F.);
#18538=ORIENTED_EDGE('',*,*,#13821,.T.);
#18539=ORIENTED_EDGE('',*,*,#13829,.F.);
#18540=ORIENTED_EDGE('',*,*,#13794,.F.);
#18541=ORIENTED_EDGE('',*,*,#13810,.F.);
#18542=ORIENTED_EDGE('',*,*,#13798,.F.);
#18543=ORIENTED_EDGE('',*,*,#13830,.F.);
#18544=ORIENTED_EDGE('',*,*,#13823,.T.);
#18545=ORIENTED_EDGE('',*,*,#13805,.F.);
#18546=ORIENTED_EDGE('',*,*,#13825,.F.);
#18547=ORIENTED_EDGE('',*,*,#13831,.F.);
#18548=ORIENTED_EDGE('',*,*,#13832,.F.);
#18549=ORIENTED_EDGE('',*,*,#13833,.F.);
#18550=ORIENTED_EDGE('',*,*,#13787,.F.);
#18551=ORIENTED_EDGE('',*,*,#13834,.F.);
#18552=ORIENTED_EDGE('',*,*,#13835,.F.);
#18553=ORIENTED_EDGE('',*,*,#13836,.F.);
#18554=ORIENTED_EDGE('',*,*,#13837,.F.);
#18555=ORIENTED_EDGE('',*,*,#13838,.T.);
#18556=ORIENTED_EDGE('',*,*,#13826,.F.);
#18557=ORIENTED_EDGE('',*,*,#13836,.T.);
#18558=ORIENTED_EDGE('',*,*,#13839,.F.);
#18559=ORIENTED_EDGE('',*,*,#13834,.T.);
#18560=ORIENTED_EDGE('',*,*,#13786,.F.);
#18561=ORIENTED_EDGE('',*,*,#13840,.T.);
#18562=ORIENTED_EDGE('',*,*,#13841,.F.);
#18563=ORIENTED_EDGE('',*,*,#13842,.F.);
#18564=ORIENTED_EDGE('',*,*,#13827,.F.);
#18565=ORIENTED_EDGE('',*,*,#13838,.F.);
#18566=ORIENTED_EDGE('',*,*,#13843,.F.);
#18567=ORIENTED_EDGE('',*,*,#13840,.F.);
#18568=ORIENTED_EDGE('',*,*,#13785,.F.);
#18569=ORIENTED_EDGE('',*,*,#13844,.F.);
#18570=ORIENTED_EDGE('',*,*,#13845,.F.);
#18571=ORIENTED_EDGE('',*,*,#13846,.F.);
#18572=ORIENTED_EDGE('',*,*,#13831,.T.);
#18573=ORIENTED_EDGE('',*,*,#13824,.F.);
#18574=ORIENTED_EDGE('',*,*,#13842,.T.);
#18575=ORIENTED_EDGE('',*,*,#13847,.F.);
#18576=ORIENTED_EDGE('',*,*,#13844,.T.);
#18577=ORIENTED_EDGE('',*,*,#13784,.F.);
#18578=ORIENTED_EDGE('',*,*,#13833,.T.);
#18579=ORIENTED_EDGE('',*,*,#13843,.T.);
#18580=ORIENTED_EDGE('',*,*,#13848,.T.);
#18581=ORIENTED_EDGE('',*,*,#13849,.F.);
#18582=ORIENTED_EDGE('',*,*,#13850,.F.);
#18583=ORIENTED_EDGE('',*,*,#13851,.F.);
#18584=ORIENTED_EDGE('',*,*,#13848,.F.);
#18585=ORIENTED_EDGE('',*,*,#13845,.T.);
#18586=ORIENTED_EDGE('',*,*,#13847,.T.);
#18587=ORIENTED_EDGE('',*,*,#13832,.T.);
#18588=ORIENTED_EDGE('',*,*,#13846,.T.);
#18589=ORIENTED_EDGE('',*,*,#13841,.T.);
#18590=ORIENTED_EDGE('',*,*,#13837,.T.);
#18591=ORIENTED_EDGE('',*,*,#13835,.T.);
#18592=ORIENTED_EDGE('',*,*,#13839,.T.);
#18593=ORIENTED_EDGE('',*,*,#13788,.F.);
#18594=ORIENTED_EDGE('',*,*,#13852,.T.);
#18595=ORIENTED_EDGE('',*,*,#13851,.T.);
#18596=ORIENTED_EDGE('',*,*,#13850,.T.);
#18597=ORIENTED_EDGE('',*,*,#13853,.T.);
#18598=ORIENTED_EDGE('',*,*,#13819,.T.);
#18599=ORIENTED_EDGE('',*,*,#13828,.T.);
#18600=ORIENTED_EDGE('',*,*,#13780,.T.);
#18601=ORIENTED_EDGE('',*,*,#13803,.T.);
#18602=ORIENTED_EDGE('',*,*,#13817,.T.);
#18603=ORIENTED_EDGE('',*,*,#13830,.T.);
#18604=ORIENTED_EDGE('',*,*,#13801,.T.);
#18605=ORIENTED_EDGE('',*,*,#13816,.T.);
#18606=ORIENTED_EDGE('',*,*,#13822,.T.);
#18607=ORIENTED_EDGE('',*,*,#13813,.T.);
#18608=ORIENTED_EDGE('',*,*,#13795,.T.);
#18609=ORIENTED_EDGE('',*,*,#13829,.T.);
#18610=ORIENTED_EDGE('',*,*,#13820,.T.);
#18611=ORIENTED_EDGE('',*,*,#13853,.F.);
#18612=ORIENTED_EDGE('',*,*,#13849,.T.);
#18613=ORIENTED_EDGE('',*,*,#13852,.F.);
#18614=ORIENTED_EDGE('',*,*,#13854,.T.);
#18615=ORIENTED_EDGE('',*,*,#13855,.T.);
#18616=ORIENTED_EDGE('',*,*,#13856,.T.);
#18617=ORIENTED_EDGE('',*,*,#13857,.T.);
#18618=ORIENTED_EDGE('',*,*,#13858,.T.);
#18619=ORIENTED_EDGE('',*,*,#13859,.T.);
#18620=ORIENTED_EDGE('',*,*,#13860,.T.);
#18621=ORIENTED_EDGE('',*,*,#13861,.T.);
#18622=ORIENTED_EDGE('',*,*,#13862,.T.);
#18623=ORIENTED_EDGE('',*,*,#13863,.T.);
#18624=ORIENTED_EDGE('',*,*,#13864,.T.);
#18625=ORIENTED_EDGE('',*,*,#13865,.T.);
#18626=ORIENTED_EDGE('',*,*,#13866,.T.);
#18627=ORIENTED_EDGE('',*,*,#13867,.T.);
#18628=ORIENTED_EDGE('',*,*,#13868,.T.);
#18629=ORIENTED_EDGE('',*,*,#13869,.T.);
#18630=ORIENTED_EDGE('',*,*,#13870,.T.);
#18631=ORIENTED_EDGE('',*,*,#13871,.T.);
#18632=ORIENTED_EDGE('',*,*,#13872,.T.);
#18633=ORIENTED_EDGE('',*,*,#13873,.T.);
#18634=ORIENTED_EDGE('',*,*,#13874,.T.);
#18635=ORIENTED_EDGE('',*,*,#13875,.T.);
#18636=ORIENTED_EDGE('',*,*,#13876,.T.);
#18637=ORIENTED_EDGE('',*,*,#13877,.T.);
#18638=ORIENTED_EDGE('',*,*,#13878,.T.);
#18639=ORIENTED_EDGE('',*,*,#13879,.T.);
#18640=ORIENTED_EDGE('',*,*,#13880,.T.);
#18641=ORIENTED_EDGE('',*,*,#13881,.T.);
#18642=ORIENTED_EDGE('',*,*,#13882,.T.);
#18643=ORIENTED_EDGE('',*,*,#13883,.T.);
#18644=ORIENTED_EDGE('',*,*,#13884,.T.);
#18645=ORIENTED_EDGE('',*,*,#13885,.T.);
#18646=ORIENTED_EDGE('',*,*,#13886,.T.);
#18647=ORIENTED_EDGE('',*,*,#13887,.T.);
#18648=ORIENTED_EDGE('',*,*,#13888,.T.);
#18649=ORIENTED_EDGE('',*,*,#13889,.T.);
#18650=ORIENTED_EDGE('',*,*,#13890,.T.);
#18651=ORIENTED_EDGE('',*,*,#13891,.T.);
#18652=ORIENTED_EDGE('',*,*,#13892,.T.);
#18653=ORIENTED_EDGE('',*,*,#13893,.T.);
#18654=ORIENTED_EDGE('',*,*,#13894,.T.);
#18655=ORIENTED_EDGE('',*,*,#13895,.T.);
#18656=ORIENTED_EDGE('',*,*,#13896,.T.);
#18657=ORIENTED_EDGE('',*,*,#13897,.T.);
#18658=ORIENTED_EDGE('',*,*,#13898,.T.);
#18659=ORIENTED_EDGE('',*,*,#13899,.T.);
#18660=ORIENTED_EDGE('',*,*,#13900,.T.);
#18661=ORIENTED_EDGE('',*,*,#13901,.T.);
#18662=ORIENTED_EDGE('',*,*,#13865,.F.);
#18663=ORIENTED_EDGE('',*,*,#13902,.F.);
#18664=ORIENTED_EDGE('',*,*,#13900,.F.);
#18665=ORIENTED_EDGE('',*,*,#13903,.T.);
#18666=ORIENTED_EDGE('',*,*,#13864,.F.);
#18667=ORIENTED_EDGE('',*,*,#13904,.F.);
#18668=ORIENTED_EDGE('',*,*,#13901,.F.);
#18669=ORIENTED_EDGE('',*,*,#13902,.T.);
#18670=ORIENTED_EDGE('',*,*,#13866,.F.);
#18671=ORIENTED_EDGE('',*,*,#13903,.F.);
#18672=ORIENTED_EDGE('',*,*,#13899,.F.);
#18673=ORIENTED_EDGE('',*,*,#13905,.T.);
#18674=ORIENTED_EDGE('',*,*,#13867,.F.);
#18675=ORIENTED_EDGE('',*,*,#13905,.F.);
#18676=ORIENTED_EDGE('',*,*,#13898,.F.);
#18677=ORIENTED_EDGE('',*,*,#13906,.T.);
#18678=ORIENTED_EDGE('',*,*,#13868,.F.);
#18679=ORIENTED_EDGE('',*,*,#13906,.F.);
#18680=ORIENTED_EDGE('',*,*,#13897,.F.);
#18681=ORIENTED_EDGE('',*,*,#13907,.T.);
#18682=ORIENTED_EDGE('',*,*,#13869,.F.);
#18683=ORIENTED_EDGE('',*,*,#13907,.F.);
#18684=ORIENTED_EDGE('',*,*,#13896,.F.);
#18685=ORIENTED_EDGE('',*,*,#13908,.T.);
#18686=ORIENTED_EDGE('',*,*,#13870,.F.);
#18687=ORIENTED_EDGE('',*,*,#13908,.F.);
#18688=ORIENTED_EDGE('',*,*,#13895,.F.);
#18689=ORIENTED_EDGE('',*,*,#13909,.T.);
#18690=ORIENTED_EDGE('',*,*,#13863,.F.);
#18691=ORIENTED_EDGE('',*,*,#13909,.F.);
#18692=ORIENTED_EDGE('',*,*,#13894,.F.);
#18693=ORIENTED_EDGE('',*,*,#13904,.T.);
#18694=ORIENTED_EDGE('',*,*,#13879,.F.);
#18695=ORIENTED_EDGE('',*,*,#13910,.F.);
#18696=ORIENTED_EDGE('',*,*,#13911,.F.);
#18697=ORIENTED_EDGE('',*,*,#13912,.T.);
#18698=ORIENTED_EDGE('',*,*,#13878,.F.);
#18699=ORIENTED_EDGE('',*,*,#13913,.F.);
#18700=ORIENTED_EDGE('',*,*,#13914,.F.);
#18701=ORIENTED_EDGE('',*,*,#13910,.T.);
#18702=ORIENTED_EDGE('',*,*,#13877,.F.);
#18703=ORIENTED_EDGE('',*,*,#13915,.F.);
#18704=ORIENTED_EDGE('',*,*,#13916,.F.);
#18705=ORIENTED_EDGE('',*,*,#13913,.T.);
#18706=ORIENTED_EDGE('',*,*,#13886,.F.);
#18707=ORIENTED_EDGE('',*,*,#13917,.F.);
#18708=ORIENTED_EDGE('',*,*,#13918,.F.);
#18709=ORIENTED_EDGE('',*,*,#13919,.T.);
#18710=ORIENTED_EDGE('',*,*,#13885,.F.);
#18711=ORIENTED_EDGE('',*,*,#13920,.F.);
#18712=ORIENTED_EDGE('',*,*,#13921,.F.);
#18713=ORIENTED_EDGE('',*,*,#13917,.T.);
#18714=ORIENTED_EDGE('',*,*,#13884,.F.);
#18715=ORIENTED_EDGE('',*,*,#13922,.F.);
#18716=ORIENTED_EDGE('',*,*,#13923,.F.);
#18717=ORIENTED_EDGE('',*,*,#13920,.T.);
#18718=ORIENTED_EDGE('',*,*,#13883,.F.);
#18719=ORIENTED_EDGE('',*,*,#13924,.F.);
#18720=ORIENTED_EDGE('',*,*,#13925,.F.);
#18721=ORIENTED_EDGE('',*,*,#13922,.T.);
#18722=ORIENTED_EDGE('',*,*,#13882,.F.);
#18723=ORIENTED_EDGE('',*,*,#13926,.F.);
#18724=ORIENTED_EDGE('',*,*,#13927,.F.);
#18725=ORIENTED_EDGE('',*,*,#13924,.T.);
#18726=ORIENTED_EDGE('',*,*,#13881,.F.);
#18727=ORIENTED_EDGE('',*,*,#13928,.F.);
#18728=ORIENTED_EDGE('',*,*,#13929,.F.);
#18729=ORIENTED_EDGE('',*,*,#13926,.T.);
#18730=ORIENTED_EDGE('',*,*,#13880,.F.);
#18731=ORIENTED_EDGE('',*,*,#13912,.F.);
#18732=ORIENTED_EDGE('',*,*,#13930,.F.);
#18733=ORIENTED_EDGE('',*,*,#13928,.T.);
#18734=ORIENTED_EDGE('',*,*,#13887,.F.);
#18735=ORIENTED_EDGE('',*,*,#13919,.F.);
#18736=ORIENTED_EDGE('',*,*,#13931,.F.);
#18737=ORIENTED_EDGE('',*,*,#13915,.T.);
#18738=ORIENTED_EDGE('',*,*,#13916,.T.);
#18739=ORIENTED_EDGE('',*,*,#13931,.T.);
#18740=ORIENTED_EDGE('',*,*,#13918,.T.);
#18741=ORIENTED_EDGE('',*,*,#13921,.T.);
#18742=ORIENTED_EDGE('',*,*,#13923,.T.);
#18743=ORIENTED_EDGE('',*,*,#13925,.T.);
#18744=ORIENTED_EDGE('',*,*,#13927,.T.);
#18745=ORIENTED_EDGE('',*,*,#13929,.T.);
#18746=ORIENTED_EDGE('',*,*,#13930,.T.);
#18747=ORIENTED_EDGE('',*,*,#13911,.T.);
#18748=ORIENTED_EDGE('',*,*,#13914,.T.);
#18749=ORIENTED_EDGE('',*,*,#13932,.T.);
#18750=ORIENTED_EDGE('',*,*,#13933,.T.);
#18751=ORIENTED_EDGE('',*,*,#13934,.T.);
#18752=ORIENTED_EDGE('',*,*,#13935,.T.);
#18753=ORIENTED_EDGE('',*,*,#13936,.T.);
#18754=ORIENTED_EDGE('',*,*,#13937,.T.);
#18755=ORIENTED_EDGE('',*,*,#13873,.F.);
#18756=ORIENTED_EDGE('',*,*,#13938,.F.);
#18757=ORIENTED_EDGE('',*,*,#13934,.F.);
#18758=ORIENTED_EDGE('',*,*,#13939,.T.);
#18759=ORIENTED_EDGE('',*,*,#13872,.F.);
#18760=ORIENTED_EDGE('',*,*,#13940,.F.);
#18761=ORIENTED_EDGE('',*,*,#13935,.F.);
#18762=ORIENTED_EDGE('',*,*,#13938,.T.);
#18763=ORIENTED_EDGE('',*,*,#13874,.F.);
#18764=ORIENTED_EDGE('',*,*,#13939,.F.);
#18765=ORIENTED_EDGE('',*,*,#13933,.F.);
#18766=ORIENTED_EDGE('',*,*,#13941,.T.);
#18767=ORIENTED_EDGE('',*,*,#13875,.F.);
#18768=ORIENTED_EDGE('',*,*,#13941,.F.);
#18769=ORIENTED_EDGE('',*,*,#13932,.F.);
#18770=ORIENTED_EDGE('',*,*,#13942,.T.);
#18771=ORIENTED_EDGE('',*,*,#13876,.F.);
#18772=ORIENTED_EDGE('',*,*,#13942,.F.);
#18773=ORIENTED_EDGE('',*,*,#13937,.F.);
#18774=ORIENTED_EDGE('',*,*,#13943,.T.);
#18775=ORIENTED_EDGE('',*,*,#13871,.F.);
#18776=ORIENTED_EDGE('',*,*,#13943,.F.);
#18777=ORIENTED_EDGE('',*,*,#13936,.F.);
#18778=ORIENTED_EDGE('',*,*,#13940,.T.);
#18779=ORIENTED_EDGE('',*,*,#13892,.F.);
#18780=ORIENTED_EDGE('',*,*,#13944,.F.);
#18781=ORIENTED_EDGE('',*,*,#13945,.F.);
#18782=ORIENTED_EDGE('',*,*,#13946,.T.);
#18783=ORIENTED_EDGE('',*,*,#13891,.F.);
#18784=ORIENTED_EDGE('',*,*,#13947,.F.);
#18785=ORIENTED_EDGE('',*,*,#13948,.F.);
#18786=ORIENTED_EDGE('',*,*,#13944,.T.);
#18787=ORIENTED_EDGE('',*,*,#13890,.F.);
#18788=ORIENTED_EDGE('',*,*,#13949,.F.);
#18789=ORIENTED_EDGE('',*,*,#13950,.F.);
#18790=ORIENTED_EDGE('',*,*,#13947,.T.);
#18791=ORIENTED_EDGE('',*,*,#13889,.F.);
#18792=ORIENTED_EDGE('',*,*,#13951,.F.);
#18793=ORIENTED_EDGE('',*,*,#13952,.F.);
#18794=ORIENTED_EDGE('',*,*,#13949,.T.);
#18795=ORIENTED_EDGE('',*,*,#13893,.F.);
#18796=ORIENTED_EDGE('',*,*,#13946,.F.);
#18797=ORIENTED_EDGE('',*,*,#13953,.F.);
#18798=ORIENTED_EDGE('',*,*,#13954,.T.);
#18799=ORIENTED_EDGE('',*,*,#13888,.F.);
#18800=ORIENTED_EDGE('',*,*,#13954,.F.);
#18801=ORIENTED_EDGE('',*,*,#13955,.F.);
#18802=ORIENTED_EDGE('',*,*,#13951,.T.);
#18803=ORIENTED_EDGE('',*,*,#13950,.T.);
#18804=ORIENTED_EDGE('',*,*,#13952,.T.);
#18805=ORIENTED_EDGE('',*,*,#13955,.T.);
#18806=ORIENTED_EDGE('',*,*,#13953,.T.);
#18807=ORIENTED_EDGE('',*,*,#13945,.T.);
#18808=ORIENTED_EDGE('',*,*,#13948,.T.);
#18809=ORIENTED_EDGE('',*,*,#13857,.F.);
#18810=ORIENTED_EDGE('',*,*,#13956,.F.);
#18811=ORIENTED_EDGE('',*,*,#13957,.F.);
#18812=ORIENTED_EDGE('',*,*,#13958,.T.);
#18813=ORIENTED_EDGE('',*,*,#13856,.F.);
#18814=ORIENTED_EDGE('',*,*,#13959,.F.);
#18815=ORIENTED_EDGE('',*,*,#13960,.F.);
#18816=ORIENTED_EDGE('',*,*,#13956,.T.);
#18817=ORIENTED_EDGE('',*,*,#13855,.F.);
#18818=ORIENTED_EDGE('',*,*,#13961,.F.);
#18819=ORIENTED_EDGE('',*,*,#13962,.F.);
#18820=ORIENTED_EDGE('',*,*,#13959,.T.);
#18821=ORIENTED_EDGE('',*,*,#13854,.F.);
#18822=ORIENTED_EDGE('',*,*,#13963,.F.);
#18823=ORIENTED_EDGE('',*,*,#13964,.F.);
#18824=ORIENTED_EDGE('',*,*,#13961,.T.);
#18825=ORIENTED_EDGE('',*,*,#13862,.F.);
#18826=ORIENTED_EDGE('',*,*,#13965,.F.);
#18827=ORIENTED_EDGE('',*,*,#13966,.F.);
#18828=ORIENTED_EDGE('',*,*,#13963,.T.);
#18829=ORIENTED_EDGE('',*,*,#13793,.F.);
#18830=ORIENTED_EDGE('',*,*,#13967,.F.);
#18831=ORIENTED_EDGE('',*,*,#13968,.F.);
#18832=ORIENTED_EDGE('',*,*,#13969,.T.);
#18833=ORIENTED_EDGE('',*,*,#13792,.F.);
#18834=ORIENTED_EDGE('',*,*,#13970,.F.);
#18835=ORIENTED_EDGE('',*,*,#13971,.F.);
#18836=ORIENTED_EDGE('',*,*,#13967,.T.);
#18837=ORIENTED_EDGE('',*,*,#13861,.F.);
#18838=ORIENTED_EDGE('',*,*,#13972,.F.);
#18839=ORIENTED_EDGE('',*,*,#13973,.F.);
#18840=ORIENTED_EDGE('',*,*,#13965,.T.);
#18841=ORIENTED_EDGE('',*,*,#13860,.F.);
#18842=ORIENTED_EDGE('',*,*,#13974,.F.);
#18843=ORIENTED_EDGE('',*,*,#13975,.F.);
#18844=ORIENTED_EDGE('',*,*,#13972,.T.);
#18845=ORIENTED_EDGE('',*,*,#13859,.F.);
#18846=ORIENTED_EDGE('',*,*,#13976,.F.);
#18847=ORIENTED_EDGE('',*,*,#13977,.F.);
#18848=ORIENTED_EDGE('',*,*,#13974,.T.);
#18849=ORIENTED_EDGE('',*,*,#13858,.F.);
#18850=ORIENTED_EDGE('',*,*,#13958,.F.);
#18851=ORIENTED_EDGE('',*,*,#13978,.F.);
#18852=ORIENTED_EDGE('',*,*,#13976,.T.);
#18853=ORIENTED_EDGE('',*,*,#13791,.F.);
#18854=ORIENTED_EDGE('',*,*,#13979,.F.);
#18855=ORIENTED_EDGE('',*,*,#13980,.F.);
#18856=ORIENTED_EDGE('',*,*,#13970,.T.);
#18857=ORIENTED_EDGE('',*,*,#13790,.F.);
#18858=ORIENTED_EDGE('',*,*,#13969,.F.);
#18859=ORIENTED_EDGE('',*,*,#13981,.F.);
#18860=ORIENTED_EDGE('',*,*,#13979,.T.);
#18861=ORIENTED_EDGE('',*,*,#13964,.T.);
#18862=ORIENTED_EDGE('',*,*,#13966,.T.);
#18863=ORIENTED_EDGE('',*,*,#13973,.T.);
#18864=ORIENTED_EDGE('',*,*,#13975,.T.);
#18865=ORIENTED_EDGE('',*,*,#13977,.T.);
#18866=ORIENTED_EDGE('',*,*,#13978,.T.);
#18867=ORIENTED_EDGE('',*,*,#13957,.T.);
#18868=ORIENTED_EDGE('',*,*,#13960,.T.);
#18869=ORIENTED_EDGE('',*,*,#13962,.T.);
#18870=ORIENTED_EDGE('',*,*,#13971,.T.);
#18871=ORIENTED_EDGE('',*,*,#13980,.T.);
#18872=ORIENTED_EDGE('',*,*,#13981,.T.);
#18873=ORIENTED_EDGE('',*,*,#13968,.T.);
#22867=CYLINDRICAL_SURFACE('',#25831,20.);
#22868=CYLINDRICAL_SURFACE('',#25843,11.5);
#22869=CYLINDRICAL_SURFACE('',#25845,12.);
#22870=CYLINDRICAL_SURFACE('',#25847,12.);
#22871=CYLINDRICAL_SURFACE('',#25849,12.);
#22872=CYLINDRICAL_SURFACE('',#25851,11.5);
#22873=CYLINDRICAL_SURFACE('',#25853,11.5);
#22874=CYLINDRICAL_SURFACE('',#25864,11.5);
#22875=CYLINDRICAL_SURFACE('',#25865,11.5);
#22876=CYLINDRICAL_SURFACE('',#25866,11.5);
#22877=CYLINDRICAL_SURFACE('',#25867,5.);
#22878=CYLINDRICAL_SURFACE('',#25877,2.1);
#22879=CYLINDRICAL_SURFACE('',#25878,20.);
#22880=CYLINDRICAL_SURFACE('',#25902,19.5);
#22881=CYLINDRICAL_SURFACE('',#25933,19.5);
#22882=CYLINDRICAL_SURFACE('',#25934,19.5);
#22883=CYLINDRICAL_SURFACE('',#25955,19.5);
#22884=CYLINDRICAL_SURFACE('',#25961,1.4361111111);
#22885=CYLINDRICAL_SURFACE('',#25972,0.4033333333);
#22886=CYLINDRICAL_SURFACE('',#25974,19.5);
#23705=ADVANCED_FACE('',(#2713),#1609,.T.);
#23706=ADVANCED_FACE('',(#2714,#1149),#1610,.T.);
#23707=ADVANCED_FACE('',(#2715),#2123,.T.);
#23708=ADVANCED_FACE('',(#2716),#22867,.T.);
#23709=ADVANCED_FACE('',(#2717),#1611,.T.);
#23710=ADVANCED_FACE('',(#2718),#1612,.T.);
#23711=ADVANCED_FACE('',(#2719),#22868,.F.);
#23712=ADVANCED_FACE('',(#2720),#22869,.F.);
#23713=ADVANCED_FACE('',(#2721),#22870,.F.);
#23714=ADVANCED_FACE('',(#2722),#22871,.F.);
#23715=ADVANCED_FACE('',(#2723),#22872,.F.);
#23716=ADVANCED_FACE('',(#2724),#22873,.F.);
#23717=ADVANCED_FACE('',(#2725,#1150),#1613,.F.);
#23718=ADVANCED_FACE('',(#2726),#22874,.F.);
#23719=ADVANCED_FACE('',(#2727),#22875,.F.);
#23720=ADVANCED_FACE('',(#2728),#22876,.F.);
#23721=ADVANCED_FACE('',(#2729),#22877,.F.);
#23722=ADVANCED_FACE('',(#2730),#1614,.T.);
#23723=ADVANCED_FACE('',(#2731),#1615,.T.);
#23724=ADVANCED_FACE('',(#2732),#1616,.F.);
#23725=ADVANCED_FACE('',(#2733),#1617,.F.);
#23726=ADVANCED_FACE('',(#2734),#1618,.T.);
#23727=ADVANCED_FACE('',(#2735),#1619,.T.);
#23728=ADVANCED_FACE('',(#2736),#22878,.F.);
#23729=ADVANCED_FACE('',(#2737,#1151,#1152,#1153,#1154,#1155),#22879,.T.);
#23730=ADVANCED_FACE('',(#2738),#22880,.T.);
#23731=ADVANCED_FACE('',(#2739),#1620,.F.);
#23732=ADVANCED_FACE('',(#2740),#1621,.F.);
#23733=ADVANCED_FACE('',(#2741),#1622,.F.);
#23734=ADVANCED_FACE('',(#2742),#1623,.F.);
#23735=ADVANCED_FACE('',(#2743),#1624,.F.);
#23736=ADVANCED_FACE('',(#2744),#1625,.F.);
#23737=ADVANCED_FACE('',(#2745),#1626,.F.);
#23738=ADVANCED_FACE('',(#2746),#1627,.F.);
#23739=ADVANCED_FACE('',(#2747),#1628,.F.);
#23740=ADVANCED_FACE('',(#2748),#1629,.F.);
#23741=ADVANCED_FACE('',(#2749),#1630,.F.);
#23742=ADVANCED_FACE('',(#2750),#1631,.F.);
#23743=ADVANCED_FACE('',(#2751),#1632,.F.);
#23744=ADVANCED_FACE('',(#2752),#1633,.F.);
#23745=ADVANCED_FACE('',(#2753),#1634,.F.);
#23746=ADVANCED_FACE('',(#2754),#1635,.F.);
#23747=ADVANCED_FACE('',(#2755),#1636,.F.);
#23748=ADVANCED_FACE('',(#2756),#1637,.F.);
#23749=ADVANCED_FACE('',(#2757),#1638,.F.);
#23750=ADVANCED_FACE('',(#2758),#22881,.T.);
#23751=ADVANCED_FACE('',(#2759),#22882,.T.);
#23752=ADVANCED_FACE('',(#2760),#1639,.F.);
#23753=ADVANCED_FACE('',(#2761),#1640,.F.);
#23754=ADVANCED_FACE('',(#2762),#1641,.F.);
#23755=ADVANCED_FACE('',(#2763),#1642,.F.);
#23756=ADVANCED_FACE('',(#2764),#1643,.F.);
#23757=ADVANCED_FACE('',(#2765),#1644,.F.);
#23758=ADVANCED_FACE('',(#2766),#1645,.F.);
#23759=ADVANCED_FACE('',(#2767),#1646,.F.);
#23760=ADVANCED_FACE('',(#2768),#1647,.F.);
#23761=ADVANCED_FACE('',(#2769),#1648,.F.);
#23762=ADVANCED_FACE('',(#2770),#1649,.F.);
#23763=ADVANCED_FACE('',(#2771),#1650,.F.);
#23764=ADVANCED_FACE('',(#2772),#22883,.T.);
#23765=ADVANCED_FACE('',(#2773),#1651,.F.);
#23766=ADVANCED_FACE('',(#2774),#1652,.F.);
#23767=ADVANCED_FACE('',(#2775),#1653,.F.);
#23768=ADVANCED_FACE('',(#2776),#22884,.F.);
#23769=ADVANCED_FACE('',(#2777),#1654,.F.);
#23770=ADVANCED_FACE('',(#2778),#1655,.T.);
#23771=ADVANCED_FACE('',(#2779),#1656,.T.);
#23772=ADVANCED_FACE('',(#2780),#1657,.F.);
#23773=ADVANCED_FACE('',(#2781),#1658,.F.);
#23774=ADVANCED_FACE('',(#2782),#1659,.F.);
#23775=ADVANCED_FACE('',(#2783),#1660,.F.);
#23776=ADVANCED_FACE('',(#2784),#22885,.T.);
#23777=ADVANCED_FACE('',(#2785),#1661,.T.);
#23778=ADVANCED_FACE('',(#2786,#1156),#22886,.T.);
#24543=CLOSED_SHELL('',(#23705,#23706,#23707,#23708,#23709,#23710,#23711,
#23712,#23713,#23714,#23715,#23716,#23717,#23718,#23719,#23720,#23721,#23722,
#23723,#23724,#23725,#23726,#23727,#23728,#23729,#23730,#23731,#23732,#23733,
#23734,#23735,#23736,#23737,#23738,#23739,#23740,#23741,#23742,#23743,#23744,
#23745,#23746,#23747,#23748,#23749,#23750,#23751,#23752,#23753,#23754,#23755,
#23756,#23757,#23758,#23759,#23760,#23761,#23762,#23763,#23764,#23765,#23766,
#23767,#23768,#23769,#23770,#23771,#23772,#23773,#23774,#23775,#23776,#23777,
#23778));
#25820=AXIS2_PLACEMENT_3D('',#52240,#29964,#29965);
#25821=AXIS2_PLACEMENT_3D('',#52241,#29966,#29967);
#25822=AXIS2_PLACEMENT_3D('',#52244,#29968,#29969);
#25823=AXIS2_PLACEMENT_3D('',#52246,#29970,#29971);
#25824=AXIS2_PLACEMENT_3D('',#52248,#29972,#29973);
#25825=AXIS2_PLACEMENT_3D('',#52249,#29974,#29975);
#25826=AXIS2_PLACEMENT_3D('',#52250,#29976,#29977);
#25827=AXIS2_PLACEMENT_3D('',#52252,#29978,#29979);
#25828=AXIS2_PLACEMENT_3D('',#52260,#29983,#29984);
#25829=AXIS2_PLACEMENT_3D('',#52261,#29985,#29986);
#25830=AXIS2_PLACEMENT_3D('',#52263,#29987,#29988);
#25831=AXIS2_PLACEMENT_3D('',#52265,#29990,#29991);
#25832=AXIS2_PLACEMENT_3D('',#52290,#29994,#29995);
#25833=AXIS2_PLACEMENT_3D('',#52291,#29996,#29997);
#25834=AXIS2_PLACEMENT_3D('',#52294,#29998,#29999);
#25835=AXIS2_PLACEMENT_3D('',#52296,#30000,#30001);
#25836=AXIS2_PLACEMENT_3D('',#52298,#30002,#30003);
#25837=AXIS2_PLACEMENT_3D('',#52299,#30004,#30005);
#25838=AXIS2_PLACEMENT_3D('',#52300,#30006,#30007);
#25839=AXIS2_PLACEMENT_3D('',#52303,#30008,#30009);
#25840=AXIS2_PLACEMENT_3D('',#52305,#30010,#30011);
#25841=AXIS2_PLACEMENT_3D('',#52307,#30012,#30013);
#25842=AXIS2_PLACEMENT_3D('',#52308,#30014,#30015);
#25843=AXIS2_PLACEMENT_3D('',#52309,#30016,#30017);
#25844=AXIS2_PLACEMENT_3D('',#52312,#30018,#30019);
#25845=AXIS2_PLACEMENT_3D('',#52315,#30022,#30023);
#25846=AXIS2_PLACEMENT_3D('',#52319,#30025,#30026);
#25847=AXIS2_PLACEMENT_3D('',#52321,#30028,#30029);
#25848=AXIS2_PLACEMENT_3D('',#52325,#30031,#30032);
#25849=AXIS2_PLACEMENT_3D('',#52327,#30034,#30035);
#25850=AXIS2_PLACEMENT_3D('',#52330,#30037,#30038);
#25851=AXIS2_PLACEMENT_3D('',#52331,#30039,#30040);
#25852=AXIS2_PLACEMENT_3D('',#52334,#30042,#30043);
#25853=AXIS2_PLACEMENT_3D('',#52335,#30044,#30045);
#25854=AXIS2_PLACEMENT_3D('',#52337,#30046,#30047);
#25855=AXIS2_PLACEMENT_3D('',#52339,#30049,#30050);
#25856=AXIS2_PLACEMENT_3D('',#52341,#30051,#30052);
#25857=AXIS2_PLACEMENT_3D('',#52343,#30053,#30054);
#25858=AXIS2_PLACEMENT_3D('',#52345,#30055,#30056);
#25859=AXIS2_PLACEMENT_3D('',#52347,#30057,#30058);
#25860=AXIS2_PLACEMENT_3D('',#52348,#30059,#30060);
#25861=AXIS2_PLACEMENT_3D('',#52349,#30061,#30062);
#25862=AXIS2_PLACEMENT_3D('',#52350,#30063,#30064);
#25863=AXIS2_PLACEMENT_3D('',#52355,#30066,#30067);
#25864=AXIS2_PLACEMENT_3D('',#52359,#30070,#30071);
#25865=AXIS2_PLACEMENT_3D('',#52361,#30073,#30074);
#25866=AXIS2_PLACEMENT_3D('',#52363,#30076,#30077);
#25867=AXIS2_PLACEMENT_3D('',#52365,#30079,#30080);
#25868=AXIS2_PLACEMENT_3D('',#52395,#30085,#30086);
#25869=AXIS2_PLACEMENT_3D('',#52399,#30089,#30090);
#25870=AXIS2_PLACEMENT_3D('',#52403,#30093,#30094);
#25871=AXIS2_PLACEMENT_3D('',#52405,#30095,#30096);
#25872=AXIS2_PLACEMENT_3D('',#52407,#30098,#30099);
#25873=AXIS2_PLACEMENT_3D('',#52409,#30100,#30101);
#25874=AXIS2_PLACEMENT_3D('',#52412,#30103,#30104);
#25875=AXIS2_PLACEMENT_3D('',#52413,#30105,#30106);
#25876=AXIS2_PLACEMENT_3D('',#52415,#30108,#30109);
#25877=AXIS2_PLACEMENT_3D('',#52417,#30111,#30112);
#25878=AXIS2_PLACEMENT_3D('',#52460,#30114,#30115);
#25879=AXIS2_PLACEMENT_3D('',#52482,#30118,#30119);
#25880=AXIS2_PLACEMENT_3D('',#52486,#30121,#30122);
#25881=AXIS2_PLACEMENT_3D('',#52490,#30124,#30125);
#25882=AXIS2_PLACEMENT_3D('',#52494,#30127,#30128);
#25883=AXIS2_PLACEMENT_3D('',#52498,#30130,#30131);
#25884=AXIS2_PLACEMENT_3D('',#52502,#30133,#30134);
#25885=AXIS2_PLACEMENT_3D('',#52506,#30136,#30137);
#25886=AXIS2_PLACEMENT_3D('',#52510,#30139,#30140);
#25887=AXIS2_PLACEMENT_3D('',#52516,#30143,#30144);
#25888=AXIS2_PLACEMENT_3D('',#52518,#30145,#30146);
#25889=AXIS2_PLACEMENT_3D('',#52522,#30148,#30149);
#25890=AXIS2_PLACEMENT_3D('',#52523,#30150,#30151);
#25891=AXIS2_PLACEMENT_3D('',#52526,#30152,#30153);
#25892=AXIS2_PLACEMENT_3D('',#52530,#30155,#30156);
#25893=AXIS2_PLACEMENT_3D('',#52532,#30157,#30158);
#25894=AXIS2_PLACEMENT_3D('',#52536,#30160,#30161);
#25895=AXIS2_PLACEMENT_3D('',#52540,#30163,#30164);
#25896=AXIS2_PLACEMENT_3D('',#52542,#30165,#30166);
#25897=AXIS2_PLACEMENT_3D('',#52545,#30168,#30169);
#25898=AXIS2_PLACEMENT_3D('',#52548,#30170,#30171);
#25899=AXIS2_PLACEMENT_3D('',#52552,#30173,#30174);
#25900=AXIS2_PLACEMENT_3D('',#52554,#30175,#30176);
#25901=AXIS2_PLACEMENT_3D('',#52557,#30178,#30179);
#25902=AXIS2_PLACEMENT_3D('',#52558,#30180,#30181);
#25903=AXIS2_PLACEMENT_3D('',#52561,#30182,#30183);
#25904=AXIS2_PLACEMENT_3D('',#52565,#30185,#30186);
#25905=AXIS2_PLACEMENT_3D('',#52569,#30188,#30189);
#25906=AXIS2_PLACEMENT_3D('',#52573,#30191,#30192);
#25907=AXIS2_PLACEMENT_3D('',#52575,#30194,#30195);
#25908=AXIS2_PLACEMENT_3D('',#52578,#30198,#30199);
#25909=AXIS2_PLACEMENT_3D('',#52580,#30201,#30202);
#25910=AXIS2_PLACEMENT_3D('',#52582,#30204,#30205);
#25911=AXIS2_PLACEMENT_3D('',#52584,#30207,#30208);
#25912=AXIS2_PLACEMENT_3D('',#52586,#30210,#30211);
#25913=AXIS2_PLACEMENT_3D('',#52588,#30213,#30214);
#25914=AXIS2_PLACEMENT_3D('',#52590,#30216,#30217);
#25915=AXIS2_PLACEMENT_3D('',#52591,#30218,#30219);
#25916=AXIS2_PLACEMENT_3D('',#52595,#30221,#30222);
#25917=AXIS2_PLACEMENT_3D('',#52597,#30224,#30225);
#25918=AXIS2_PLACEMENT_3D('',#52601,#30228,#30229);
#25919=AXIS2_PLACEMENT_3D('',#52604,#30231,#30232);
#25920=AXIS2_PLACEMENT_3D('',#52605,#30233,#30234);
#25921=AXIS2_PLACEMENT_3D('',#52611,#30238,#30239);
#25922=AXIS2_PLACEMENT_3D('',#52614,#30241,#30242);
#25923=AXIS2_PLACEMENT_3D('',#52615,#30243,#30244);
#25924=AXIS2_PLACEMENT_3D('',#52618,#30246,#30247);
#25925=AXIS2_PLACEMENT_3D('',#52619,#30248,#30249);
#25926=AXIS2_PLACEMENT_3D('',#52623,#30252,#30253);
#25927=AXIS2_PLACEMENT_3D('',#52626,#30255,#30256);
#25928=AXIS2_PLACEMENT_3D('',#52627,#30257,#30258);
#25929=AXIS2_PLACEMENT_3D('',#52631,#30261,#30262);
#25930=AXIS2_PLACEMENT_3D('',#52632,#30263,#30264);
#25931=AXIS2_PLACEMENT_3D('',#52633,#30265,#30266);
#25932=AXIS2_PLACEMENT_3D('',#52634,#30267,#30268);
#25933=AXIS2_PLACEMENT_3D('',#52635,#30269,#30270);
#25934=AXIS2_PLACEMENT_3D('',#52636,#30271,#30272);
#25935=AXIS2_PLACEMENT_3D('',#52639,#30273,#30274);
#25936=AXIS2_PLACEMENT_3D('',#52643,#30276,#30277);
#25937=AXIS2_PLACEMENT_3D('',#52645,#30278,#30279);
#25938=AXIS2_PLACEMENT_3D('',#52648,#30281,#30282);
#25939=AXIS2_PLACEMENT_3D('',#52649,#30283,#30284);
#25940=AXIS2_PLACEMENT_3D('',#52652,#30287,#30288);
#25941=AXIS2_PLACEMENT_3D('',#52654,#30290,#30291);
#25942=AXIS2_PLACEMENT_3D('',#52656,#30293,#30294);
#25943=AXIS2_PLACEMENT_3D('',#52658,#30296,#30297);
#25944=AXIS2_PLACEMENT_3D('',#52660,#30299,#30300);
#25945=AXIS2_PLACEMENT_3D('',#52661,#30301,#30302);
#25946=AXIS2_PLACEMENT_3D('',#52667,#30306,#30307);
#25947=AXIS2_PLACEMENT_3D('',#52670,#30309,#30310);
#25948=AXIS2_PLACEMENT_3D('',#52671,#30311,#30312);
#25949=AXIS2_PLACEMENT_3D('',#52674,#30314,#30315);
#25950=AXIS2_PLACEMENT_3D('',#52675,#30316,#30317);
#25951=AXIS2_PLACEMENT_3D('',#52679,#30320,#30321);
#25952=AXIS2_PLACEMENT_3D('',#52681,#30322,#30323);
#25953=AXIS2_PLACEMENT_3D('',#52683,#30325,#30326);
#25954=AXIS2_PLACEMENT_3D('',#52684,#30327,#30328);
#25955=AXIS2_PLACEMENT_3D('',#52685,#30329,#30330);
#25956=AXIS2_PLACEMENT_3D('',#52686,#30331,#30332);
#25957=AXIS2_PLACEMENT_3D('',#52690,#30334,#30335);
#25958=AXIS2_PLACEMENT_3D('',#52692,#30337,#30338);
#25959=AXIS2_PLACEMENT_3D('',#52696,#30341,#30342);
#25960=AXIS2_PLACEMENT_3D('',#52699,#30344,#30345);
#25961=AXIS2_PLACEMENT_3D('',#52700,#30346,#30347);
#25962=AXIS2_PLACEMENT_3D('',#52719,#30349,#30350);
#25963=AXIS2_PLACEMENT_3D('',#52723,#30353,#30354);
#25964=AXIS2_PLACEMENT_3D('',#52727,#30356,#30357);
#25965=AXIS2_PLACEMENT_3D('',#52729,#30359,#30360);
#25966=AXIS2_PLACEMENT_3D('',#52733,#30363,#30364);
#25967=AXIS2_PLACEMENT_3D('',#52736,#30366,#30367);
#25968=AXIS2_PLACEMENT_3D('',#52737,#30368,#30369);
#25969=AXIS2_PLACEMENT_3D('',#52741,#30372,#30373);
#25970=AXIS2_PLACEMENT_3D('',#52744,#30375,#30376);
#25971=AXIS2_PLACEMENT_3D('',#52745,#30377,#30378);
#25972=AXIS2_PLACEMENT_3D('',#52747,#30380,#30381);
#25973=AXIS2_PLACEMENT_3D('',#52768,#30383,#30384);
#25974=AXIS2_PLACEMENT_3D('',#52770,#30386,#30387);
#29964=DIRECTION('axis',(0.,0.,1.));
#29965=DIRECTION('refdir',(1.,0.,0.));
#29966=DIRECTION('center_axis',(1.,0.,0.));
#29967=DIRECTION('ref_axis',(0.,1.,0.));
#29968=DIRECTION('center_axis',(-1.,0.,0.));
#29969=DIRECTION('ref_axis',(0.,-0.499999999993262,-0.866025403788329));
#29970=DIRECTION('center_axis',(-1.,0.,0.));
#29971=DIRECTION('ref_axis',(0.,0.,1.));
#29972=DIRECTION('center_axis',(-1.,0.,0.));
#29973=DIRECTION('ref_axis',(0.,1.,0.));
#29974=DIRECTION('center_axis',(-1.,0.,0.));
#29975=DIRECTION('ref_axis',(0.,0.,-1.));
#29976=DIRECTION('center_axis',(-1.,0.,0.));
#29977=DIRECTION('ref_axis',(0.,0.,1.));
#29978=DIRECTION('center_axis',(-1.,0.,0.));
#29979=DIRECTION('ref_axis',(0.,0.,1.));
#29980=DIRECTION('',(0.,0.,-1.));
#29981=DIRECTION('',(0.,1.,0.));
#29982=DIRECTION('',(0.,0.,1.));
#29983=DIRECTION('center_axis',(1.,0.,0.));
#29984=DIRECTION('ref_axis',(0.,0.,1.));
#29985=DIRECTION('center_axis',(1.,0.,0.));
#29986=DIRECTION('ref_axis',(0.,0.,1.));
#29987=DIRECTION('center_axis',(-1.,0.,0.));
#29988=DIRECTION('ref_axis',(0.,0.,1.));
#29989=DIRECTION('',(-0.707106781186548,-8.65956056235493E-17,0.707106781186547));
#29990=DIRECTION('center_axis',(-1.,0.,0.));
#29991=DIRECTION('ref_axis',(0.,0.,1.));
#29992=DIRECTION('',(-1.,0.,0.));
#29993=DIRECTION('',(1.,0.,0.));
#29994=DIRECTION('center_axis',(-1.,0.,0.));
#29995=DIRECTION('ref_axis',(0.,0.,1.));
#29996=DIRECTION('center_axis',(1.,0.,0.));
#29997=DIRECTION('ref_axis',(0.,1.,0.));
#29998=DIRECTION('center_axis',(-1.,0.,0.));
#29999=DIRECTION('ref_axis',(0.,1.,0.));
#30000=DIRECTION('center_axis',(-1.,0.,0.));
#30001=DIRECTION('ref_axis',(0.,0.,1.));
#30002=DIRECTION('center_axis',(-1.,0.,0.));
#30003=DIRECTION('ref_axis',(0.,-0.499999999993262,0.866025403788329));
#30004=DIRECTION('center_axis',(-1.,0.,0.));
#30005=DIRECTION('ref_axis',(0.,0.,-1.));
#30006=DIRECTION('center_axis',(1.,0.,0.));
#30007=DIRECTION('ref_axis',(0.,1.,0.));
#30008=DIRECTION('center_axis',(-1.,0.,0.));
#30009=DIRECTION('ref_axis',(0.,-0.499999999993262,-0.866025403788329));
#30010=DIRECTION('center_axis',(-1.,0.,0.));
#30011=DIRECTION('ref_axis',(0.,0.,-1.));
#30012=DIRECTION('center_axis',(-1.,0.,0.));
#30013=DIRECTION('ref_axis',(0.,-0.499999999993262,0.866025403788329));
#30014=DIRECTION('center_axis',(-1.,0.,0.));
#30015=DIRECTION('ref_axis',(0.,0.,1.));
#30016=DIRECTION('center_axis',(1.,0.,0.));
#30017=DIRECTION('ref_axis',(0.,-0.499999999993262,-0.866025403788329));
#30018=DIRECTION('center_axis',(-1.,0.,0.));
#30019=DIRECTION('ref_axis',(0.,-0.499999999993262,-0.866025403788329));
#30020=DIRECTION('',(-1.,0.,0.));
#30021=DIRECTION('',(1.,0.,0.));
#30022=DIRECTION('center_axis',(1.,0.,0.));
#30023=DIRECTION('ref_axis',(0.,1.22464679914735E-16,1.));
#30024=DIRECTION('',(-1.,0.,0.));
#30025=DIRECTION('center_axis',(-1.,0.,0.));
#30026=DIRECTION('ref_axis',(0.,0.,-1.));
#30027=DIRECTION('',(1.,0.,0.));
#30028=DIRECTION('center_axis',(1.,0.,0.));
#30029=DIRECTION('ref_axis',(0.,0.,-1.));
#30030=DIRECTION('',(-1.,0.,0.));
#30031=DIRECTION('center_axis',(-1.,0.,0.));
#30032=DIRECTION('ref_axis',(0.,0.,-1.));
#30033=DIRECTION('',(1.,0.,0.));
#30034=DIRECTION('center_axis',(1.,0.,0.));
#30035=DIRECTION('ref_axis',(0.,0.,-1.));
#30036=DIRECTION('',(-1.,0.,0.));
#30037=DIRECTION('center_axis',(-1.,0.,0.));
#30038=DIRECTION('ref_axis',(0.,0.,-1.));
#30039=DIRECTION('center_axis',(1.,0.,0.));
#30040=DIRECTION('ref_axis',(0.,0.17575598334211,-0.98443376329718));
#30041=DIRECTION('',(1.,0.,0.));
#30042=DIRECTION('center_axis',(-1.,0.,0.));
#30043=DIRECTION('ref_axis',(0.,-0.499999999993262,0.866025403788329));
#30044=DIRECTION('center_axis',(1.,0.,0.));
#30045=DIRECTION('ref_axis',(0.,-0.499999999993262,0.866025403788329));
#30046=DIRECTION('center_axis',(-1.,0.,0.));
#30047=DIRECTION('ref_axis',(0.,-0.499999999993262,0.866025403788329));
#30048=DIRECTION('',(-1.,0.,0.));
#30049=DIRECTION('center_axis',(-1.,0.,0.));
#30050=DIRECTION('ref_axis',(0.,0.,1.));
#30051=DIRECTION('center_axis',(-1.,0.,0.));
#30052=DIRECTION('ref_axis',(0.,0.,1.));
#30053=DIRECTION('center_axis',(-1.,0.,0.));
#30054=DIRECTION('ref_axis',(0.,1.,0.));
#30055=DIRECTION('center_axis',(-1.,0.,0.));
#30056=DIRECTION('ref_axis',(0.,0.,1.));
#30057=DIRECTION('center_axis',(-1.,0.,0.));
#30058=DIRECTION('ref_axis',(0.,0.,1.));
#30059=DIRECTION('center_axis',(-1.,0.,0.));
#30060=DIRECTION('ref_axis',(0.,1.,0.));
#30061=DIRECTION('center_axis',(-1.,0.,0.));
#30062=DIRECTION('ref_axis',(0.,0.,1.));
#30063=DIRECTION('center_axis',(-1.,0.,0.));
#30064=DIRECTION('ref_axis',(0.,-0.499999999993262,-0.866025403788329));
#30065=DIRECTION('',(0.,0.,1.));
#30066=DIRECTION('center_axis',(-1.,0.,0.));
#30067=DIRECTION('ref_axis',(0.,0.,1.));
#30068=DIRECTION('',(0.,0.,-1.));
#30069=DIRECTION('',(0.,-1.,0.));
#30070=DIRECTION('center_axis',(1.,0.,0.));
#30071=DIRECTION('ref_axis',(0.,-0.94042263903113,0.340007735202781));
#30072=DIRECTION('',(1.,0.,0.));
#30073=DIRECTION('center_axis',(1.,0.,0.));
#30074=DIRECTION('ref_axis',(0.,1.,0.));
#30075=DIRECTION('',(-1.,0.,0.));
#30076=DIRECTION('center_axis',(1.,0.,0.));
#30077=DIRECTION('ref_axis',(0.,0.764666655685446,0.644426028092314));
#30078=DIRECTION('',(1.,0.,0.));
#30079=DIRECTION('center_axis',(-1.,0.,0.));
#30080=DIRECTION('ref_axis',(0.,0.,1.));
#30081=DIRECTION('',(1.,0.,0.));
#30082=DIRECTION('',(1.,0.,0.));
#30083=DIRECTION('',(-1.,0.,0.));
#30084=DIRECTION('',(-1.,0.,0.));
#30085=DIRECTION('center_axis',(0.,-1.,0.));
#30086=DIRECTION('ref_axis',(0.,0.,-1.));
#30087=DIRECTION('',(0.,0.,1.));
#30088=DIRECTION('',(1.,0.,0.));
#30089=DIRECTION('center_axis',(0.,-1.,0.));
#30090=DIRECTION('ref_axis',(0.,0.,-1.));
#30091=DIRECTION('',(0.,0.,-1.));
#30092=DIRECTION('',(1.,0.,0.));
#30093=DIRECTION('center_axis',(0.,0.,-1.));
#30094=DIRECTION('ref_axis',(0.,-1.,0.));
#30095=DIRECTION('center_axis',(0.,0.,1.));
#30096=DIRECTION('ref_axis',(1.,0.,0.));
#30097=DIRECTION('',(-1.,0.,0.));
#30098=DIRECTION('center_axis',(0.,0.,-1.));
#30099=DIRECTION('ref_axis',(0.,-1.,0.));
#30100=DIRECTION('center_axis',(0.,0.,1.));
#30101=DIRECTION('ref_axis',(1.,0.,0.));
#30102=DIRECTION('',(-1.,0.,0.));
#30103=DIRECTION('center_axis',(0.,0.,1.));
#30104=DIRECTION('ref_axis',(1.,0.,0.));
#30105=DIRECTION('center_axis',(0.,1.,0.));
#30106=DIRECTION('ref_axis',(1.,0.,0.));
#30107=DIRECTION('',(0.,0.,-1.));
#30108=DIRECTION('center_axis',(0.,1.,0.));
#30109=DIRECTION('ref_axis',(1.,0.,0.));
#30110=DIRECTION('',(0.,0.,1.));
#30111=DIRECTION('center_axis',(0.,0.,-1.));
#30112=DIRECTION('ref_axis',(1.,0.,0.));
#30113=DIRECTION('',(0.,0.,-1.));
#30114=DIRECTION('center_axis',(-1.,0.,0.));
#30115=DIRECTION('ref_axis',(0.,0.,1.));
#30116=DIRECTION('',(1.,0.,0.));
#30117=DIRECTION('',(1.,0.,0.));
#30118=DIRECTION('center_axis',(-0.946028810149232,-0.324082536350894,-7.74377105026033E-10));
#30119=DIRECTION('ref_axis',(-0.0328036819517733,0.0957571728004204,0.994864052173802));
#30120=DIRECTION('',(1.,0.,0.));
#30121=DIRECTION('center_axis',(0.94602881016076,0.324082536317243,-7.10771293430115E-14));
#30122=DIRECTION('ref_axis',(-0.0103965438556825,0.03034853443635,0.999485306712121));
#30123=DIRECTION('',(1.,0.,0.));
#30124=DIRECTION('center_axis',(-1.,0.,0.));
#30125=DIRECTION('ref_axis',(0.,0.,1.));
#30126=DIRECTION('',(1.,0.,0.));
#30127=DIRECTION('center_axis',(1.,0.,0.));
#30128=DIRECTION('ref_axis',(0.,0.,1.));
#30129=DIRECTION('',(-1.,0.,0.));
#30130=DIRECTION('center_axis',(-1.,0.,0.));
#30131=DIRECTION('ref_axis',(0.,0.,1.));
#30132=DIRECTION('',(1.,0.,0.));
#30133=DIRECTION('center_axis',(1.,0.,0.));
#30134=DIRECTION('ref_axis',(0.,0.,1.));
#30135=DIRECTION('',(1.,0.,0.));
#30136=DIRECTION('center_axis',(1.,0.,0.));
#30137=DIRECTION('ref_axis',(0.,0.,1.));
#30138=DIRECTION('',(-1.,0.,0.));
#30139=DIRECTION('center_axis',(-1.,0.,0.));
#30140=DIRECTION('ref_axis',(0.,0.,1.));
#30141=DIRECTION('',(1.,0.,0.));
#30142=DIRECTION('',(-1.,0.,0.));
#30143=DIRECTION('center_axis',(-0.50000000001139,-0.866025403777863,-5.6567377117582E-14));
#30144=DIRECTION('ref_axis',(0.866025403777863,-0.50000000001139,-7.49337626227376E-11));
#30145=DIRECTION('center_axis',(0.500000000011408,-0.866025403777852,1.85864239100662E-13));
#30146=DIRECTION('ref_axis',(0.866025403777852,0.500000000011408,-4.16431008826601E-10));
#30147=DIRECTION('',(-1.,0.,0.));
#30148=DIRECTION('center_axis',(-0.500000000001134,0.866025403783784,5.52352953831563E-15));
#30149=DIRECTION('ref_axis',(0.866025403783784,0.500000000001134,-1.60186152837855E-11));
#30150=DIRECTION('center_axis',(0.500000000001135,0.866025403783783,-5.52352953831541E-15));
#30151=DIRECTION('ref_axis',(0.866025403783783,-0.500000000001135,-3.15235664736174E-11));
#30152=DIRECTION('center_axis',(0.855183382509445,0.518325556267202,0.));
#30153=DIRECTION('ref_axis',(-0.518325556267202,0.855183382509445,0.));
#30154=DIRECTION('',(1.,0.,0.));
#30155=DIRECTION('center_axis',(0.855183382508501,0.518325556268759,0.));
#30156=DIRECTION('ref_axis',(-0.518325556268759,0.855183382508501,0.));
#30157=DIRECTION('center_axis',(-1.,0.,0.));
#30158=DIRECTION('ref_axis',(0.,0.,1.));
#30159=DIRECTION('',(1.,0.,0.));
#30160=DIRECTION('center_axis',(1.,0.,0.));
#30161=DIRECTION('ref_axis',(0.,0.,1.));
#30162=DIRECTION('',(-1.,0.,0.));
#30163=DIRECTION('center_axis',(-1.,0.,0.));
#30164=DIRECTION('ref_axis',(0.,0.,1.));
#30165=DIRECTION('center_axis',(0.829037572548639,-0.55919290348024,0.));
#30166=DIRECTION('ref_axis',(0.55919290348024,0.829037572548639,0.));
#30167=DIRECTION('',(-1.,0.,0.));
#30168=DIRECTION('center_axis',(-0.82903757255312,0.559192903473596,0.));
#30169=DIRECTION('ref_axis',(0.559192903473596,0.82903757255312,0.));
#30170=DIRECTION('center_axis',(-0.500000000011392,0.866025403777861,-2.42431616218218E-14));
#30171=DIRECTION('ref_axis',(0.866025403777861,0.500000000011392,1.34504687835035E-10));
#30172=DIRECTION('',(1.,0.,0.));
#30173=DIRECTION('center_axis',(0.500000000001136,-0.866025403783783,-8.28529430747307E-15));
#30174=DIRECTION('ref_axis',(0.866025403783783,0.500000000001136,-3.29777777975133E-11));
#30175=DIRECTION('center_axis',(-0.500000000001135,-0.866025403783783,-5.5235295383155E-15));
#30176=DIRECTION('ref_axis',(0.866025403783783,-0.500000000001135,-1.55386342491463E-11));
#30177=DIRECTION('',(1.,0.,0.));
#30178=DIRECTION('center_axis',(0.50000000001139,0.866025403777863,-4.84863232436438E-14));
#30179=DIRECTION('ref_axis',(0.866025403777863,-0.50000000001139,-3.46934311402352E-10));
#30180=DIRECTION('center_axis',(-1.,0.,0.));
#30181=DIRECTION('ref_axis',(0.,0.,1.));
#30182=DIRECTION('center_axis',(1.,0.,0.));
#30183=DIRECTION('ref_axis',(0.,0.,1.));
#30184=DIRECTION('',(-1.,0.,0.));
#30185=DIRECTION('center_axis',(1.,0.,0.));
#30186=DIRECTION('ref_axis',(0.,0.,1.));
#30187=DIRECTION('',(1.,0.,0.));
#30188=DIRECTION('center_axis',(-1.,0.,0.));
#30189=DIRECTION('ref_axis',(0.,0.,1.));
#30190=DIRECTION('',(-1.,0.,0.));
#30191=DIRECTION('center_axis',(-1.,0.,0.));
#30192=DIRECTION('ref_axis',(0.,0.,1.));
#30193=DIRECTION('',(-1.,0.,0.));
#30194=DIRECTION('center_axis',(1.,0.,0.));
#30195=DIRECTION('ref_axis',(0.,1.,0.));
#30196=DIRECTION('',(0.,0.,1.));
#30197=DIRECTION('',(0.,0.,1.));
#30198=DIRECTION('center_axis',(0.,1.,0.));
#30199=DIRECTION('ref_axis',(1.,0.,0.));
#30200=DIRECTION('',(0.,0.,1.));
#30201=DIRECTION('center_axis',(0.,1.,0.));
#30202=DIRECTION('ref_axis',(1.,0.,0.));
#30203=DIRECTION('',(0.,0.,1.));
#30204=DIRECTION('center_axis',(1.,0.,0.));
#30205=DIRECTION('ref_axis',(0.,1.,0.));
#30206=DIRECTION('',(0.,0.,1.));
#30207=DIRECTION('center_axis',(0.,-1.,0.));
#30208=DIRECTION('ref_axis',(0.,0.,-1.));
#30209=DIRECTION('',(0.,0.,1.));
#30210=DIRECTION('center_axis',(-1.,0.,0.));
#30211=DIRECTION('ref_axis',(0.,0.,1.));
#30212=DIRECTION('',(0.,0.,1.));
#30213=DIRECTION('center_axis',(0.,1.,0.));
#30214=DIRECTION('ref_axis',(1.,0.,0.));
#30215=DIRECTION('',(0.,0.,1.));
#30216=DIRECTION('center_axis',(-1.,0.,0.));
#30217=DIRECTION('ref_axis',(0.,0.,1.));
#30218=DIRECTION('center_axis',(0.855183382508501,0.518325556268759,0.));
#30219=DIRECTION('ref_axis',(0.,0.,-1.));
#30220=DIRECTION('',(0.,0.,1.));
#30221=DIRECTION('center_axis',(-0.855183382508501,-0.518325556268759,0.));
#30222=DIRECTION('ref_axis',(-0.518325556268759,0.855183382508501,0.));
#30223=DIRECTION('',(0.,0.,1.));
#30224=DIRECTION('center_axis',(0.,1.,0.));
#30225=DIRECTION('ref_axis',(1.,0.,0.));
#30226=DIRECTION('',(0.,0.,1.));
#30227=DIRECTION('',(-1.,0.,0.));
#30228=DIRECTION('center_axis',(-0.855183382509445,-0.518325556267202,0.));
#30229=DIRECTION('ref_axis',(-0.518325556267202,0.855183382509445,0.));
#30230=DIRECTION('',(0.,0.,1.));
#30231=DIRECTION('center_axis',(-0.855183382509445,-0.518325556267202,0.));
#30232=DIRECTION('ref_axis',(-0.518325556267202,0.855183382509445,0.));
#30233=DIRECTION('center_axis',(0.,-1.,0.));
#30234=DIRECTION('ref_axis',(0.,0.,-1.));
#30235=DIRECTION('',(0.,0.,1.));
#30236=DIRECTION('',(1.,0.,0.));
#30237=DIRECTION('',(0.,0.,1.));
#30238=DIRECTION('center_axis',(0.829037572548639,-0.55919290348024,0.));
#30239=DIRECTION('ref_axis',(0.,0.,-1.));
#30240=DIRECTION('',(0.,0.,1.));
#30241=DIRECTION('center_axis',(-0.829037572548639,0.55919290348024,0.));
#30242=DIRECTION('ref_axis',(0.55919290348024,0.829037572548639,0.));
#30243=DIRECTION('center_axis',(-1.,0.,0.));
#30244=DIRECTION('ref_axis',(0.,0.,1.));
#30245=DIRECTION('',(0.,0.,1.));
#30246=DIRECTION('center_axis',(1.,0.,0.));
#30247=DIRECTION('ref_axis',(0.,0.,1.));
#30248=DIRECTION('center_axis',(0.,-1.,0.));
#30249=DIRECTION('ref_axis',(0.,0.,-1.));
#30250=DIRECTION('',(0.,0.,1.));
#30251=DIRECTION('',(1.,0.,0.));
#30252=DIRECTION('center_axis',(1.,0.,0.));
#30253=DIRECTION('ref_axis',(0.,1.,0.));
#30254=DIRECTION('',(0.,0.,1.));
#30255=DIRECTION('center_axis',(-1.,0.,0.));
#30256=DIRECTION('ref_axis',(0.,0.,1.));
#30257=DIRECTION('center_axis',(0.,1.,0.));
#30258=DIRECTION('ref_axis',(1.,0.,0.));
#30259=DIRECTION('',(0.,0.,1.));
#30260=DIRECTION('',(-1.,0.,0.));
#30261=DIRECTION('center_axis',(-1.,0.,0.));
#30262=DIRECTION('ref_axis',(0.,0.,1.));
#30263=DIRECTION('center_axis',(1.,0.,0.));
#30264=DIRECTION('ref_axis',(0.,0.,1.));
#30265=DIRECTION('center_axis',(-0.82903757255312,0.559192903473596,0.));
#30266=DIRECTION('ref_axis',(0.,0.,1.));
#30267=DIRECTION('center_axis',(0.82903757255312,-0.559192903473596,0.));
#30268=DIRECTION('ref_axis',(0.559192903473596,0.82903757255312,0.));
#30269=DIRECTION('center_axis',(-1.,0.,0.));
#30270=DIRECTION('ref_axis',(0.,0.,1.));
#30271=DIRECTION('center_axis',(-1.,0.,0.));
#30272=DIRECTION('ref_axis',(0.,0.,1.));
#30273=DIRECTION('center_axis',(0.500000000001133,-0.866025403783785,-1.87875446695563E-14));
#30274=DIRECTION('ref_axis',(0.866025403783785,0.500000000001133,1.73760906682291E-11));
#30275=DIRECTION('',(1.,0.,0.));
#30276=DIRECTION('center_axis',(-0.500000000011412,0.86602540377785,-2.35812383115421E-13));
#30277=DIRECTION('ref_axis',(0.86602540377785,0.500000000011412,4.13106356090107E-10));
#30278=DIRECTION('center_axis',(0.500000000011409,0.866025403777852,-1.88649906492394E-13));
#30279=DIRECTION('ref_axis',(0.866025403777852,-0.500000000011409,-1.71455444984074E-12));
#30280=DIRECTION('',(1.,0.,0.));
#30281=DIRECTION('center_axis',(-0.500000000001134,-0.866025403783784,-2.6839349527939E-15));
#30282=DIRECTION('ref_axis',(0.866025403783784,-0.500000000001134,2.2215382786634E-11));
#30283=DIRECTION('center_axis',(0.500000000011394,-0.866025403777861,0.));
#30284=DIRECTION('ref_axis',(0.,0.,-1.));
#30285=DIRECTION('',(0.,0.,1.));
#30286=DIRECTION('',(0.,0.,1.));
#30287=DIRECTION('center_axis',(-0.500000000011394,-0.866025403777861,0.));
#30288=DIRECTION('ref_axis',(-0.866025403777861,0.500000000011394,0.));
#30289=DIRECTION('',(0.,0.,1.));
#30290=DIRECTION('center_axis',(0.,-1.,0.));
#30291=DIRECTION('ref_axis',(0.,0.,-1.));
#30292=DIRECTION('',(0.,0.,1.));
#30293=DIRECTION('center_axis',(-0.500000000001135,0.866025403783784,0.));
#30294=DIRECTION('ref_axis',(0.,0.,1.));
#30295=DIRECTION('',(0.,0.,1.));
#30296=DIRECTION('center_axis',(0.500000000001135,0.866025403783784,0.));
#30297=DIRECTION('ref_axis',(0.,0.,-1.));
#30298=DIRECTION('',(0.,0.,1.));
#30299=DIRECTION('center_axis',(0.,-1.,0.));
#30300=DIRECTION('ref_axis',(0.,0.,-1.));
#30301=DIRECTION('center_axis',(0.,1.,0.));
#30302=DIRECTION('ref_axis',(1.,0.,0.));
#30303=DIRECTION('',(0.,0.,1.));
#30304=DIRECTION('',(-1.,0.,0.));
#30305=DIRECTION('',(0.,0.,1.));
#30306=DIRECTION('center_axis',(-0.500000000001135,-0.866025403783784,0.));
#30307=DIRECTION('ref_axis',(-0.866025403783784,0.500000000001135,0.));
#30308=DIRECTION('',(0.,0.,1.));
#30309=DIRECTION('center_axis',(0.500000000001134,0.866025403783784,-1.34196747639693E-14));
#30310=DIRECTION('ref_axis',(0.866025403783784,-0.500000000001134,-2.93336016297228E-11));
#30311=DIRECTION('center_axis',(0.500000000001135,-0.866025403783784,0.));
#30312=DIRECTION('ref_axis',(0.,0.,-1.));
#30313=DIRECTION('',(0.,0.,1.));
#30314=DIRECTION('center_axis',(-0.500000000001132,0.866025403783785,-2.41554145751436E-14));
#30315=DIRECTION('ref_axis',(0.866025403783785,0.500000000001132,1.58006467766065E-11));
#30316=DIRECTION('center_axis',(0.,1.,0.));
#30317=DIRECTION('ref_axis',(1.,0.,0.));
#30318=DIRECTION('',(0.,0.,1.));
#30319=DIRECTION('',(-1.,0.,0.));
#30320=DIRECTION('center_axis',(0.500000000011394,0.866025403777861,0.));
#30321=DIRECTION('ref_axis',(0.,0.,-1.));
#30322=DIRECTION('center_axis',(-0.500000000011412,-0.86602540377785,-2.35812383115473E-13));
#30323=DIRECTION('ref_axis',(0.86602540377785,-0.500000000011412,1.59264985720823E-10));
#30324=DIRECTION('',(0.,0.,1.));
#30325=DIRECTION('center_axis',(-0.500000000011394,0.866025403777861,0.));
#30326=DIRECTION('ref_axis',(0.,0.,1.));
#30327=DIRECTION('center_axis',(0.500000000011402,-0.866025403777856,-1.17906191557739E-13));
#30328=DIRECTION('ref_axis',(0.866025403777856,0.500000000011402,-2.60506588040655E-10));
#30329=DIRECTION('center_axis',(-1.,0.,0.));
#30330=DIRECTION('ref_axis',(0.,0.,1.));
#30331=DIRECTION('center_axis',(0.946028810160758,0.324082536317247,0.));
#30332=DIRECTION('ref_axis',(0.,0.,-1.));
#30333=DIRECTION('',(0.,0.,1.));
#30334=DIRECTION('center_axis',(-0.94602881016076,-0.324082536317242,7.53842350672448E-14));
#30335=DIRECTION('ref_axis',(-0.033646559749939,0.0982176184129628,0.99459600263136));
#30336=DIRECTION('',(0.,0.,1.));
#30337=DIRECTION('center_axis',(0.,1.,0.));
#30338=DIRECTION('ref_axis',(1.,0.,0.));
#30339=DIRECTION('',(0.,0.,1.));
#30340=DIRECTION('',(-1.,0.,0.));
#30341=DIRECTION('center_axis',(-0.946028810171404,-0.324082536286173,0.));
#30342=DIRECTION('ref_axis',(-0.324082536286173,0.946028810171404,0.));
#30343=DIRECTION('',(0.,0.,1.));
#30344=DIRECTION('center_axis',(0.946028810149238,0.324082536350876,7.54583899480575E-10));
#30345=DIRECTION('ref_axis',(-0.00721450072149016,0.0210598351143057,0.999752186456373));
#30346=DIRECTION('center_axis',(0.,0.,1.));
#30347=DIRECTION('ref_axis',(-0.587785252292473,0.809016994374947,0.));
#30348=DIRECTION('',(0.,0.,1.));
#30349=DIRECTION('center_axis',(0.,-1.,0.));
#30350=DIRECTION('ref_axis',(0.,0.,-1.));
#30351=DIRECTION('',(0.,0.,1.));
#30352=DIRECTION('',(1.,0.,0.));
#30353=DIRECTION('center_axis',(1.,0.,0.));
#30354=DIRECTION('ref_axis',(0.,1.,0.));
#30355=DIRECTION('',(0.,0.,1.));
#30356=DIRECTION('center_axis',(1.,0.,0.));
#30357=DIRECTION('ref_axis',(0.,0.,1.));
#30358=DIRECTION('',(0.,0.,1.));
#30359=DIRECTION('center_axis',(0.,-1.,0.));
#30360=DIRECTION('ref_axis',(0.,0.,-1.));
#30361=DIRECTION('',(0.,0.,1.));
#30362=DIRECTION('',(-1.,0.,0.));
#30363=DIRECTION('center_axis',(1.,0.,0.));
#30364=DIRECTION('ref_axis',(0.,1.,0.));
#30365=DIRECTION('',(0.,0.,1.));
#30366=DIRECTION('center_axis',(-1.,0.,0.));
#30367=DIRECTION('ref_axis',(0.,0.,1.));
#30368=DIRECTION('center_axis',(0.,1.,0.));
#30369=DIRECTION('ref_axis',(1.,0.,0.));
#30370=DIRECTION('',(0.,0.,1.));
#30371=DIRECTION('',(-1.,0.,0.));
#30372=DIRECTION('center_axis',(-1.,0.,0.));
#30373=DIRECTION('ref_axis',(0.,0.,1.));
#30374=DIRECTION('',(0.,0.,1.));
#30375=DIRECTION('center_axis',(1.,0.,0.));
#30376=DIRECTION('ref_axis',(0.,0.,1.));
#30377=DIRECTION('center_axis',(0.,1.,0.));
#30378=DIRECTION('ref_axis',(1.,0.,0.));
#30379=DIRECTION('',(-1.,0.,0.));
#30380=DIRECTION('center_axis',(0.,0.,1.));
#30381=DIRECTION('ref_axis',(0.,1.,0.));
#30382=DIRECTION('',(0.,0.,1.));
#30383=DIRECTION('center_axis',(0.,1.,0.));
#30384=DIRECTION('ref_axis',(1.,0.,0.));
#30385=DIRECTION('',(1.,0.,0.));
#30386=DIRECTION('center_axis',(-1.,0.,0.));
#30387=DIRECTION('ref_axis',(0.,0.,1.));
#52240=CARTESIAN_POINT('',(0.,0.,0.));
#52241=CARTESIAN_POINT('Origin',(6.,0.,10.));
#52242=CARTESIAN_POINT('',(6.,-11.5470739757602,-3.26574380475891));
#52243=CARTESIAN_POINT('',(6.,-19.921468401738,-1.77062043322529));
#52244=CARTESIAN_POINT('Origin',(6.,-13.8564064606,8.));
#52245=CARTESIAN_POINT('',(6.,-11.4941364764755,-16.3671875));
#52246=CARTESIAN_POINT('Origin',(6.,0.,0.));
#52247=CARTESIAN_POINT('',(6.,-8.60175408505985,-8.3671875));
#52248=CARTESIAN_POINT('Origin',(6.,0.,-16.));
#52249=CARTESIAN_POINT('Origin',(6.,0.,0.));
#52250=CARTESIAN_POINT('Origin',(-33.,0.,9.5));
#52251=CARTESIAN_POINT('',(-33.,2.32682891837997E-15,-19.));
#52252=CARTESIAN_POINT('Origin',(-33.,0.,0.));
#52253=CARTESIAN_POINT('',(-33.,-1.5,-4.76969600708473));
#52254=CARTESIAN_POINT('',(-33.,-1.5,-6.4));
#52255=CARTESIAN_POINT('',(-33.,-1.5,3.15));
#52256=CARTESIAN_POINT('',(-33.,1.5,-6.4));
#52257=CARTESIAN_POINT('',(-33.,0.,-6.4));
#52258=CARTESIAN_POINT('',(-33.,1.5,-4.76969600708473));
#52259=CARTESIAN_POINT('',(-33.,1.5,3.15));
#52260=CARTESIAN_POINT('Origin',(-33.,0.,0.));
#52261=CARTESIAN_POINT('Origin',(-32.5,0.,0.));
#52262=CARTESIAN_POINT('',(-32.,2.44929359829471E-15,-20.));
#52263=CARTESIAN_POINT('Origin',(-32.,0.,0.));
#52264=CARTESIAN_POINT('',(-32.5,2.38806125833734E-15,-19.5));
#52265=CARTESIAN_POINT('Origin',(-13.,0.,0.));
#52266=CARTESIAN_POINT('',(-3.7202200813,-0.2994444445,19.9977581999748));
#52267=CARTESIAN_POINT('',(-4.3435534146,-0.2994444445,19.9977581999748));
#52268=CARTESIAN_POINT('',(-4.03188674795,-0.2994444445,19.9977581999748));
#52269=CARTESIAN_POINT('',(-4.3435534146,-1.1061111111,19.969389530226));
#52270=CARTESIAN_POINT('Ctrl Pts',(-4.3435534146,-0.2994444445,19.9977581999748));
#52271=CARTESIAN_POINT('Ctrl Pts',(-4.39419529583398,-0.2994444445,19.9977581999748));
#52272=CARTESIAN_POINT('Ctrl Pts',(-4.44821240138141,-0.309565031449933,
19.9976146851541));
#52273=CARTESIAN_POINT('Ctrl Pts',(-4.54758041279513,-0.350722737591021,
19.9969351943239));
#52274=CARTESIAN_POINT('Ctrl Pts',(-4.59293124895252,-0.381759842781414,
19.9963882206146));
#52275=CARTESIAN_POINT('Ctrl Pts',(-4.66456114163788,-0.453382333903515,
19.994892548385));
#52276=CARTESIAN_POINT('Ctrl Pts',(-4.69560697302298,-0.498746314496724,
19.993842130762));
#52277=CARTESIAN_POINT('Ctrl Pts',(-4.73676959169473,-0.5981279615852,19.9911158762495));
#52278=CARTESIAN_POINT('Ctrl Pts',(-4.7468867479,-0.652145173345914,19.9894290439444));
#52279=CARTESIAN_POINT('Ctrl Pts',(-4.7468867479,-0.753438288963382,19.9858675169476));
#52280=CARTESIAN_POINT('Ctrl Pts',(-4.73675961734101,-0.80746838265751,
19.9837551246746));
#52281=CARTESIAN_POINT('Ctrl Pts',(-4.69558023913546,-0.906857064706403,
19.9794915935354));
#52282=CARTESIAN_POINT('Ctrl Pts',(-4.66452814741898,-0.952216188266304,
19.9773514320566));
#52283=CARTESIAN_POINT('Ctrl Pts',(-4.59290252845076,-1.02381445280548,
19.9738100392531));
#52284=CARTESIAN_POINT('Ctrl Pts',(-4.54756443095206,-1.05484068319396,
19.9721740344373));
#52285=CARTESIAN_POINT('Ctrl Pts',(-4.44821243395584,-1.09598926486806,
19.9699582388217));
#52286=CARTESIAN_POINT('Ctrl Pts',(-4.39419807843,-1.1061111111,19.969389530226));
#52287=CARTESIAN_POINT('Ctrl Pts',(-4.3435534146,-1.1061111111,19.969389530226));
#52288=CARTESIAN_POINT('',(-3.7202200813,-1.1061111111,19.969389530226));
#52289=CARTESIAN_POINT('',(-4.03188674795,-1.1061111111,19.969389530226));
#52290=CARTESIAN_POINT('Origin',(-3.7202200813,0.,0.));
#52291=CARTESIAN_POINT('Origin',(6.,0.,10.));
#52292=CARTESIAN_POINT('',(6.,8.60175408505985,-8.3671875));
#52293=CARTESIAN_POINT('',(6.,11.4941364764755,-16.3671875));
#52294=CARTESIAN_POINT('Origin',(6.,0.,-16.));
#52295=CARTESIAN_POINT('',(6.,19.921468401738,-1.77062043322529));
#52296=CARTESIAN_POINT('Origin',(6.,0.,0.));
#52297=CARTESIAN_POINT('',(6.,11.5470739757602,-3.26574380475891));
#52298=CARTESIAN_POINT('Origin',(6.,13.8564064606,8.));
#52299=CARTESIAN_POINT('Origin',(6.,0.,0.));
#52300=CARTESIAN_POINT('Origin',(6.,0.,10.));
#52301=CARTESIAN_POINT('',(6.,-8.42733192529161,18.1378079331809));
#52302=CARTESIAN_POINT('',(6.,-2.94531989074286,11.632931304757));
#52303=CARTESIAN_POINT('Origin',(6.,-13.8564064606,8.));
#52304=CARTESIAN_POINT('',(6.,2.94531989074286,11.632931304757));
#52305=CARTESIAN_POINT('Origin',(6.,0.,0.));
#52306=CARTESIAN_POINT('',(6.,8.42733192529161,18.1378079331809));
#52307=CARTESIAN_POINT('Origin',(6.,13.8564064606,8.));
#52308=CARTESIAN_POINT('Origin',(6.,0.,0.));
#52309=CARTESIAN_POINT('Origin',(-1.,-13.8564064606,8.));
#52310=CARTESIAN_POINT('',(-8.,-11.5470739757602,-3.26574380475891));
#52311=CARTESIAN_POINT('',(-8.,-19.921468401738,-1.77062043322529));
#52312=CARTESIAN_POINT('Origin',(-8.,-13.8564064606,8.));
#52313=CARTESIAN_POINT('',(-1.,-19.921468401738,-1.77062043322529));
#52314=CARTESIAN_POINT('',(-1.,-11.5470739757602,-3.26574380475891));
#52315=CARTESIAN_POINT('Origin',(-1.,0.,0.));
#52316=CARTESIAN_POINT('',(-8.,-2.94531989074286,11.632931304757));
#52317=CARTESIAN_POINT('',(-1.,-2.94531989074286,11.632931304757));
#52318=CARTESIAN_POINT('',(-8.,2.94531989074286,11.632931304757));
#52319=CARTESIAN_POINT('Origin',(-8.,0.,0.));
#52320=CARTESIAN_POINT('',(-1.,2.94531989074286,11.632931304757));
#52321=CARTESIAN_POINT('Origin',(-1.,0.,0.));
#52322=CARTESIAN_POINT('',(-8.,11.5470739757602,-3.26574380475891));
#52323=CARTESIAN_POINT('',(-1.,11.5470739757602,-3.26574380475891));
#52324=CARTESIAN_POINT('',(-8.,8.60175408505985,-8.3671875));
#52325=CARTESIAN_POINT('Origin',(-8.,0.,0.));
#52326=CARTESIAN_POINT('',(-1.,8.60175408505985,-8.3671875));
#52327=CARTESIAN_POINT('Origin',(-1.,0.,0.));
#52328=CARTESIAN_POINT('',(-8.,-8.60175408505985,-8.3671875));
#52329=CARTESIAN_POINT('',(-1.,-8.60175408505985,-8.3671875));
#52330=CARTESIAN_POINT('Origin',(-8.,0.,0.));
#52331=CARTESIAN_POINT('Origin',(-1.,13.8564064606,8.));
#52332=CARTESIAN_POINT('',(-8.,19.921468401738,-1.77062043322529));
#52333=CARTESIAN_POINT('',(-1.,19.921468401738,-1.77062043322529));
#52334=CARTESIAN_POINT('Origin',(-8.,13.8564064606,8.));
#52335=CARTESIAN_POINT('Origin',(-1.,13.8564064606,8.));
#52336=CARTESIAN_POINT('',(-8.,8.42733192529161,18.1378079331809));
#52337=CARTESIAN_POINT('Origin',(-8.,13.8564064606,8.));
#52338=CARTESIAN_POINT('',(-1.,8.42733192529161,18.1378079331809));
#52339=CARTESIAN_POINT('Origin',(-8.,13.8564064606,8.));
#52340=CARTESIAN_POINT('',(-8.,-8.42733192529161,18.1378079331809));
#52341=CARTESIAN_POINT('Origin',(-8.,0.,0.));
#52342=CARTESIAN_POINT('',(-8.,-11.4941364764755,-16.3671875));
#52343=CARTESIAN_POINT('Origin',(-8.,0.,-16.));
#52344=CARTESIAN_POINT('',(-8.,-2.44929359829471E-15,-20.));
#52345=CARTESIAN_POINT('Origin',(-8.,0.,0.));
#52346=CARTESIAN_POINT('',(-8.,11.4941364764755,-16.3671875));
#52347=CARTESIAN_POINT('Origin',(-8.,0.,0.));
#52348=CARTESIAN_POINT('Origin',(-8.,0.,-16.));
#52349=CARTESIAN_POINT('Origin',(-8.,0.,0.));
#52350=CARTESIAN_POINT('Origin',(-8.,-13.8564064606,8.));
#52351=CARTESIAN_POINT('',(-8.,-1.5,-6.4));
#52352=CARTESIAN_POINT('',(-8.,-1.5,-4.76969600708473));
#52353=CARTESIAN_POINT('',(-8.,-1.5,2.4));
#52354=CARTESIAN_POINT('',(-8.,1.5,-4.76969600708473));
#52355=CARTESIAN_POINT('Origin',(-8.,0.,0.));
#52356=CARTESIAN_POINT('',(-8.,1.5,-6.4));
#52357=CARTESIAN_POINT('',(-8.,1.5,2.4));
#52358=CARTESIAN_POINT('',(-8.,6.9282032303,-6.4));
#52359=CARTESIAN_POINT('Origin',(-1.,0.,-16.));
#52360=CARTESIAN_POINT('',(-1.,-11.4941364764755,-16.3671875));
#52361=CARTESIAN_POINT('Origin',(-1.,0.,-16.));
#52362=CARTESIAN_POINT('',(-1.,11.4941364764755,-16.3671875));
#52363=CARTESIAN_POINT('Origin',(-1.,-13.8564064606,8.));
#52364=CARTESIAN_POINT('',(-1.,-8.42733192529161,18.1378079331809));
#52365=CARTESIAN_POINT('Origin',(-20.5,0.,0.));
#52366=CARTESIAN_POINT('',(-21.5303061543301,-1.5,-4.76969600708473));
#52367=CARTESIAN_POINT('',(-20.5,-1.5,-4.76969600708473));
#52368=CARTESIAN_POINT('',(-24.4696938456699,-1.5,-4.76969600708473));
#52369=CARTESIAN_POINT('Ctrl Pts',(-24.4696938456699,-1.5,-4.76969600708473));
#52370=CARTESIAN_POINT('Ctrl Pts',(-24.2875078566679,-1.67850508453567,
-4.71355875506578));
#52371=CARTESIAN_POINT('Ctrl Pts',(-24.0592673499683,-1.83355795563958,
-4.65305931877349));
#52372=CARTESIAN_POINT('Ctrl Pts',(-23.5501354824849,-2.04585962054866,
-4.56378013142765));
#52373=CARTESIAN_POINT('Ctrl Pts',(-23.2674916717861,-2.1,-4.53762052181537));
#52374=CARTESIAN_POINT('Ctrl Pts',(-23.,-2.1,-4.53762052181537));
#52375=CARTESIAN_POINT('Ctrl Pts',(-22.7325083282139,-2.1,-4.53762052181537));
#52376=CARTESIAN_POINT('Ctrl Pts',(-22.4498645175151,-2.04585962054866,
-4.56378013142765));
#52377=CARTESIAN_POINT('Ctrl Pts',(-21.9407326500317,-1.83355795563958,
-4.65305931877349));
#52378=CARTESIAN_POINT('Ctrl Pts',(-21.7124921433321,-1.67850508453567,
-4.71355875506578));
#52379=CARTESIAN_POINT('Ctrl Pts',(-21.5303061543301,-1.5,-4.76969600708473));
#52380=CARTESIAN_POINT('',(-20.5,-1.5,-4.76969600708473));
#52381=CARTESIAN_POINT('',(-24.4696938456699,1.5,-4.76969600708473));
#52382=CARTESIAN_POINT('',(-20.5,1.5,-4.76969600708473));
#52383=CARTESIAN_POINT('',(-21.5303061543301,1.5,-4.76969600708473));
#52384=CARTESIAN_POINT('Ctrl Pts',(-21.5303061543301,1.5,-4.76969600708473));
#52385=CARTESIAN_POINT('Ctrl Pts',(-21.7124921433321,1.67850508453567,-4.71355875506578));
#52386=CARTESIAN_POINT('Ctrl Pts',(-21.9407326500317,1.83355795563958,-4.65305931877349));
#52387=CARTESIAN_POINT('Ctrl Pts',(-22.4498645175151,2.04585962054866,-4.56378013142765));
#52388=CARTESIAN_POINT('Ctrl Pts',(-22.7325083282139,2.1,-4.53762052181537));
#52389=CARTESIAN_POINT('Ctrl Pts',(-23.2674916717861,2.1,-4.53762052181537));
#52390=CARTESIAN_POINT('Ctrl Pts',(-23.5501354824849,2.04585962054866,-4.56378013142765));
#52391=CARTESIAN_POINT('Ctrl Pts',(-24.0592673499683,1.83355795563958,-4.65305931877349));
#52392=CARTESIAN_POINT('Ctrl Pts',(-24.2875078566679,1.67850508453567,-4.71355875506578));
#52393=CARTESIAN_POINT('Ctrl Pts',(-24.4696938456699,1.5,-4.76969600708473));
#52394=CARTESIAN_POINT('',(-20.5,1.5,-4.76969600708473));
#52395=CARTESIAN_POINT('Origin',(-20.5,1.5,-3.2));
#52396=CARTESIAN_POINT('',(-21.5303061543301,1.5,-6.4));
#52397=CARTESIAN_POINT('',(-21.5303061543301,1.5,-5.58484800354236));
#52398=CARTESIAN_POINT('',(-20.5,1.5,-6.4));
#52399=CARTESIAN_POINT('Origin',(-20.5,1.5,-3.2));
#52400=CARTESIAN_POINT('',(-24.4696938456699,1.5,-6.4));
#52401=CARTESIAN_POINT('',(-24.4696938456699,1.5,-5.58484800354236));
#52402=CARTESIAN_POINT('',(-20.5,1.5,-6.4));
#52403=CARTESIAN_POINT('Origin',(-20.5,0.,-6.4));
#52404=CARTESIAN_POINT('',(-21.5303061543301,-1.5,-6.4));
#52405=CARTESIAN_POINT('Origin',(-23.,0.,-6.4));
#52406=CARTESIAN_POINT('',(-20.5,-1.5,-6.4));
#52407=CARTESIAN_POINT('Origin',(-20.5,0.,-6.4));
#52408=CARTESIAN_POINT('',(-25.1,2.57175827820944E-16,-6.4));
#52409=CARTESIAN_POINT('Origin',(-23.,0.,-6.4));
#52410=CARTESIAN_POINT('',(-24.4696938456699,-1.5,-6.4));
#52411=CARTESIAN_POINT('',(-20.5,-1.5,-6.4));
#52412=CARTESIAN_POINT('Origin',(-23.,0.,-6.4));
#52413=CARTESIAN_POINT('Origin',(-20.5,-1.5,-3.2));
#52414=CARTESIAN_POINT('',(-21.5303061543301,-1.5,-5.58484800354236));
#52415=CARTESIAN_POINT('Origin',(-20.5,-1.5,-3.2));
#52416=CARTESIAN_POINT('',(-24.4696938456699,-1.5,-5.58484800354236));
#52417=CARTESIAN_POINT('Origin',(-23.,0.,-10.));
#52418=CARTESIAN_POINT('',(-25.1,2.57175827820944E-16,-20.));
#52419=CARTESIAN_POINT('',(-25.1,2.57175827820944E-16,-10.));
#52420=CARTESIAN_POINT('',(-20.9,0.,-20.));
#52421=CARTESIAN_POINT('Ctrl Pts',(-20.9,4.16333634234434E-16,-20.));
#52422=CARTESIAN_POINT('Ctrl Pts',(-20.9,0.263888990751172,-20.));
#52423=CARTESIAN_POINT('Ctrl Pts',(-20.9527780741314,0.545235237847868,
-19.9942425936951));
#52424=CARTESIAN_POINT('Ctrl Pts',(-21.1671514943451,1.06257490219278,-19.97343117591));
#52425=CARTESIAN_POINT('Ctrl Pts',(-21.3287361087815,1.29858458976497,-19.9586721250997));
#52426=CARTESIAN_POINT('Ctrl Pts',(-21.7014161819223,1.67126466290584,-19.9309254589373));
#52427=CARTESIAN_POINT('Ctrl Pts',(-21.9374255317885,1.83284867450471,-19.9161307432363));
#52428=CARTESIAN_POINT('Ctrl Pts',(-22.4547640622183,2.04722164681422,-19.8952376620524));
#52429=CARTESIAN_POINT('Ctrl Pts',(-22.7361099164069,2.1,-19.8894444366855));
#52430=CARTESIAN_POINT('Ctrl Pts',(-23.2638900835931,2.1,-19.8894444366855));
#52431=CARTESIAN_POINT('Ctrl Pts',(-23.5452359377817,2.04722164681422,-19.8952376620524));
#52432=CARTESIAN_POINT('Ctrl Pts',(-24.0625744682115,1.83284867450471,-19.9161307432363));
#52433=CARTESIAN_POINT('Ctrl Pts',(-24.2985838180777,1.67126466290584,-19.9309254589373));
#52434=CARTESIAN_POINT('Ctrl Pts',(-24.6712638912185,1.29858458976497,-19.9586721250997));
#52435=CARTESIAN_POINT('Ctrl Pts',(-24.8328485056549,1.06257490219277,-19.97343117591));
#52436=CARTESIAN_POINT('Ctrl Pts',(-25.0472219258686,0.545235237847867,
-19.9942425936951));
#52437=CARTESIAN_POINT('Ctrl Pts',(-25.1,0.263888990751172,-20.));
#52438=CARTESIAN_POINT('Ctrl Pts',(-25.1,-6.93889390390723E-17,-20.));
#52439=CARTESIAN_POINT('',(-23.,-2.1,-19.8894444366855));
#52440=CARTESIAN_POINT('Ctrl Pts',(-23.,-2.1,-19.8894444366855));
#52441=CARTESIAN_POINT('Ctrl Pts',(-22.7361099164069,-2.1,-19.8894444366855));
#52442=CARTESIAN_POINT('Ctrl Pts',(-22.4547640622183,-2.04722164681422,
-19.8952376620524));
#52443=CARTESIAN_POINT('Ctrl Pts',(-21.9374255317885,-1.83284867450471,
-19.9161307432363));
#52444=CARTESIAN_POINT('Ctrl Pts',(-21.7014161819223,-1.67126466290584,
-19.9309254589373));
#52445=CARTESIAN_POINT('Ctrl Pts',(-21.3287361087815,-1.29858458976497,
-19.9586721250997));
#52446=CARTESIAN_POINT('Ctrl Pts',(-21.1671514943451,-1.06257490219277,
-19.97343117591));
#52447=CARTESIAN_POINT('Ctrl Pts',(-20.9527780741314,-0.545235237847867,
-19.9942425936951));
#52448=CARTESIAN_POINT('Ctrl Pts',(-20.9,-0.263888990751171,-20.));
#52449=CARTESIAN_POINT('Ctrl Pts',(-20.9,-5.20417042793042E-17,-20.));
#52450=CARTESIAN_POINT('Ctrl Pts',(-25.1,-3.46944695195361E-16,-20.));
#52451=CARTESIAN_POINT('Ctrl Pts',(-25.1,-0.263888990751172,-20.));
#52452=CARTESIAN_POINT('Ctrl Pts',(-25.0472219258686,-0.545235237847867,
-19.9942425936951));
#52453=CARTESIAN_POINT('Ctrl Pts',(-24.8328485056549,-1.06257490219277,
-19.97343117591));
#52454=CARTESIAN_POINT('Ctrl Pts',(-24.6712638912185,-1.29858458976497,
-19.9586721250997));
#52455=CARTESIAN_POINT('Ctrl Pts',(-24.2985838180777,-1.67126466290584,
-19.9309254589373));
#52456=CARTESIAN_POINT('Ctrl Pts',(-24.0625744682115,-1.83284867450471,
-19.9161307432363));
#52457=CARTESIAN_POINT('Ctrl Pts',(-23.5452359377817,-2.04722164681422,
-19.8952376620524));
#52458=CARTESIAN_POINT('Ctrl Pts',(-23.2638900835931,-2.1,-19.8894444366855));
#52459=CARTESIAN_POINT('Ctrl Pts',(-23.,-2.1,-19.8894444366855));
#52460=CARTESIAN_POINT('Origin',(-13.,0.,0.));
#52461=CARTESIAN_POINT('',(-13.,-2.44929359829471E-15,-20.));
#52462=CARTESIAN_POINT('',(-13.,-2.44929359829471E-15,-20.));
#52463=CARTESIAN_POINT('',(-4.3435534146,-2.1388888889,19.8852999555184));
#52464=CARTESIAN_POINT('',(-5.18767834635794,0.459060516890588,19.9947308919583));
#52465=CARTESIAN_POINT('Ctrl Pts',(-5.18767834635794,0.459060516890587,
19.9947308919583));
#52466=CARTESIAN_POINT('Ctrl Pts',(-5.24968129137097,0.414012740477042,
19.9957651472147));
#52467=CARTESIAN_POINT('Ctrl Pts',(-5.30716488138641,0.364591710747686,
19.9967442102515));
#52468=CARTESIAN_POINT('Ctrl Pts',(-5.48665323742873,0.185057927007366,
19.9995504652193));
#52469=CARTESIAN_POINT('Ctrl Pts',(-5.59715741138799,0.0235509943668747,
20.0007685496482));
#52470=CARTESIAN_POINT('Ctrl Pts',(-5.7436627884403,-0.330259044510279,
19.9980555602176));
#52471=CARTESIAN_POINT('Ctrl Pts',(-5.7796645257,-0.522560848653025,19.993985306904));
#52472=CARTESIAN_POINT('Ctrl Pts',(-5.7796645257,-0.883349185014401,19.9812997715422));
#52473=CARTESIAN_POINT('Ctrl Pts',(-5.74353603624199,-1.07581469312434,
19.971831595325));
#52474=CARTESIAN_POINT('Ctrl Pts',(-5.59681775573534,-1.4297140658822,19.9496203526915));
#52475=CARTESIAN_POINT('Ctrl Pts',(-5.48623409908571,-1.59115913013439,
19.9370154287515));
#52476=CARTESIAN_POINT('Ctrl Pts',(-5.23128841814184,-1.84591622773468,
19.9150423979699));
#52477=CARTESIAN_POINT('Ctrl Pts',(-5.06995436664432,-1.95632911293912,
19.9042256075891));
#52478=CARTESIAN_POINT('Ctrl Pts',(-4.71629161866783,-2.10281902804406,
19.8892828626319));
#52479=CARTESIAN_POINT('Ctrl Pts',(-4.52395392331701,-2.1388888889,19.8852999555184));
#52480=CARTESIAN_POINT('Ctrl Pts',(-4.3435534146,-2.1388888889,19.8852999555184));
#52481=CARTESIAN_POINT('',(-5.7631397208,2.1388888889,19.8852999555184));
#52482=CARTESIAN_POINT('Origin',(-5.03059422324816,0.0005165593435702,-2.33120559308216));
#52483=CARTESIAN_POINT('',(-4.7295794663,2.1388888889,19.8852999555184));
#52484=CARTESIAN_POINT('',(-5.24635959355,2.1388888889,19.8852999555184));
#52485=CARTESIAN_POINT('',(-4.2292347159,0.6783333333,19.9884932871123));
#52486=CARTESIAN_POINT('Origin',(-3.99709194624176,0.000685748014040422,
-2.32885472330861));
#52487=CARTESIAN_POINT('',(-3.7202200813,0.6783333333,19.9884932871123));
#52488=CARTESIAN_POINT('',(-3.9747273986,0.6783333333,19.9884932871123));
#52489=CARTESIAN_POINT('',(-3.7202200813,2.1388888889,19.8852999555184));
#52490=CARTESIAN_POINT('Origin',(-3.7202200813,0.,0.));
#52491=CARTESIAN_POINT('',(-2.7424423035,2.1388888889,19.8852999555184));
#52492=CARTESIAN_POINT('',(-3.2313311924,2.1388888889,19.8852999555184));
#52493=CARTESIAN_POINT('',(-2.7424423035,-2.1388888889,19.8852999555184));
#52494=CARTESIAN_POINT('Origin',(-2.7424423035,0.,0.));
#52495=CARTESIAN_POINT('',(-3.54299785905,-2.1388888889,19.8852999555184));
#52496=CARTESIAN_POINT('',(-1.4888888889,-1.1611111111,19.9662670769395));
#52497=CARTESIAN_POINT('',(-1.4888888889,2.1388888889,19.8852999555184));
#52498=CARTESIAN_POINT('Origin',(-1.4888888889,0.,0.));
#52499=CARTESIAN_POINT('',(-0.5111111111,2.1388888889,19.8852999555184));
#52500=CARTESIAN_POINT('',(-1.,2.1388888889,19.8852999555184));
#52501=CARTESIAN_POINT('',(-0.5111111111,-1.1611111111,19.9662670769395));
#52502=CARTESIAN_POINT('Origin',(-0.5111111111,0.,0.));
#52503=CARTESIAN_POINT('',(0.5277777778,-1.1611111111,19.9662670769395));
#52504=CARTESIAN_POINT('',(0.00833333335000042,-1.1611111111,19.9662670769395));
#52505=CARTESIAN_POINT('',(0.5277777778,-2.1388888889,19.8852999555184));
#52506=CARTESIAN_POINT('Origin',(0.527777777800001,0.,0.));
#52507=CARTESIAN_POINT('',(-2.5277777778,-2.1388888889,19.8852999555184));
#52508=CARTESIAN_POINT('',(-1.,-2.1388888889,19.8852999555184));
#52509=CARTESIAN_POINT('',(-2.5277777778,-1.1611111111,19.9662670769395));
#52510=CARTESIAN_POINT('Origin',(-2.5277777778,0.,0.));
#52511=CARTESIAN_POINT('',(-2.00833333335,-1.1611111111,19.9662670769395));
#52512=CARTESIAN_POINT('',(3.7631397208,2.75,19.8100353356575));
#52513=CARTESIAN_POINT('',(1.8075841652,2.75,19.8100353356575));
#52514=CARTESIAN_POINT('',(2.785361943,2.75,19.8100353356575));
#52515=CARTESIAN_POINT('',(-1.,4.3709594736,19.5165241085637));
#52516=CARTESIAN_POINT('Origin',(6.57072388981035,-2.27381335982102E-9,
-1.34364674941878E-8));
#52517=CARTESIAN_POINT('',(-3.8075841652,2.75,19.8100353356575));
#52518=CARTESIAN_POINT('Origin',(-8.5707238638722,1.26959015522843E-8,6.91637080940666E-8));
#52519=CARTESIAN_POINT('',(-5.7631397208,2.75,19.8100353356575));
#52520=CARTESIAN_POINT('',(-4.785361943,2.75,19.8100353356575));
#52521=CARTESIAN_POINT('',(-1.,5.5,19.2288845230294));
#52522=CARTESIAN_POINT('Origin',(-10.526279440744,4.94369545300799E-10,
2.25620633287349E-9));
#52523=CARTESIAN_POINT('Origin',(8.52627944326717,-9.62673274429449E-10,
-4.51972903547926E-9));
#52524=CARTESIAN_POINT('',(1.9747474276,-0.2016666667,19.9989832380434));
#52525=CARTESIAN_POINT('',(0.5561396937,2.1388888889,19.8852999555184));
#52526=CARTESIAN_POINT('Origin',(1.85251751839491,0.,0.));
#52527=CARTESIAN_POINT('',(1.6994942043,2.1388888889,19.8852999555184));
#52528=CARTESIAN_POINT('',(1.127816949,2.1388888889,19.8852999555184));
#52529=CARTESIAN_POINT('',(2.785361943,0.3473197978,19.9969839965445));
#52530=CARTESIAN_POINT('Origin',(2.99587202900023,0.,0.));
#52531=CARTESIAN_POINT('',(2.785361943,2.1388888889,19.8852999555184));
#52532=CARTESIAN_POINT('Origin',(2.785361943,0.,0.));
#52533=CARTESIAN_POINT('',(3.7631397208,2.1388888889,19.8852999555184));
#52534=CARTESIAN_POINT('',(3.2742508319,2.1388888889,19.8852999555184));
#52535=CARTESIAN_POINT('',(3.7631397208,-2.1388888889,19.8852999555184));
#52536=CARTESIAN_POINT('Origin',(3.7631397208,0.,0.));
#52537=CARTESIAN_POINT('',(2.785361943,-2.1388888889,19.8852999555184));
#52538=CARTESIAN_POINT('',(3.2742508319,-2.1388888889,19.8852999555184));
#52539=CARTESIAN_POINT('',(2.785361943,-0.7484330612,19.9859912927256));
#52540=CARTESIAN_POINT('Origin',(2.785361943,0.,0.));
#52541=CARTESIAN_POINT('',(1.8474876449,-2.1388888889,19.8852999555184));
#52542=CARTESIAN_POINT('Origin',(3.29018641707832,0.,0.));
#52543=CARTESIAN_POINT('',(0.6680745397,-2.1388888889,19.8852999555184));
#52544=CARTESIAN_POINT('',(1.2577810923,-2.1388888889,19.8852999555184));
#52545=CARTESIAN_POINT('Origin',(2.11077331185338,0.,0.));
#52546=CARTESIAN_POINT('',(-1.,-4.3709594736,19.5165241085637));
#52547=CARTESIAN_POINT('',(1.8075841652,-2.75,19.8100353356575));
#52548=CARTESIAN_POINT('Origin',(6.57072387874695,-4.11288225699025E-9,
2.09971195985759E-8));
#52549=CARTESIAN_POINT('',(3.7631397208,-2.75,19.8100353356575));
#52550=CARTESIAN_POINT('',(2.785361943,-2.75,19.8100353356575));
#52551=CARTESIAN_POINT('',(-1.,-5.5,19.2288845230294));
#52552=CARTESIAN_POINT('Origin',(8.52627944334428,1.00725594531781E-9,-4.7267834091258E-9));
#52553=CARTESIAN_POINT('',(-5.7631397208,-2.75,19.8100353356575));
#52554=CARTESIAN_POINT('Origin',(-10.5262794407692,-4.79505324335605E-10,
2.19413154312065E-9));
#52555=CARTESIAN_POINT('',(-3.8075841652,-2.75,19.8100353356575));
#52556=CARTESIAN_POINT('',(-4.785361943,-2.75,19.8100353356575));
#52557=CARTESIAN_POINT('Origin',(-8.57072386754017,-1.05836966968198E-8,
5.72841307722172E-8));
#52558=CARTESIAN_POINT('Origin',(-1.,0.,0.));
#52559=CARTESIAN_POINT('',(-1.4888888889,2.1388888889,19.3823413013222));
#52560=CARTESIAN_POINT('',(-1.4888888889,-1.1611111111,19.4654006120521));
#52561=CARTESIAN_POINT('Origin',(-1.4888888889,0.,0.));
#52562=CARTESIAN_POINT('',(-2.5277777778,-1.1611111111,19.4654006120521));
#52563=CARTESIAN_POINT('',(-2.00833333335,-1.1611111111,19.4654006120521));
#52564=CARTESIAN_POINT('',(-2.5277777778,-2.1388888889,19.3823413013222));
#52565=CARTESIAN_POINT('Origin',(-2.5277777778,0.,0.));
#52566=CARTESIAN_POINT('',(0.5277777778,-2.1388888889,19.3823413013222));
#52567=CARTESIAN_POINT('',(-1.,-2.1388888889,19.3823413013222));
#52568=CARTESIAN_POINT('',(0.5277777778,-1.1611111111,19.4654006120521));
#52569=CARTESIAN_POINT('Origin',(0.5277777778,0.,0.));
#52570=CARTESIAN_POINT('',(-0.5111111111,-1.1611111111,19.4654006120521));
#52571=CARTESIAN_POINT('',(0.00833333334999997,-1.1611111111,19.4654006120521));
#52572=CARTESIAN_POINT('',(-0.5111111111,2.1388888889,19.3823413013222));
#52573=CARTESIAN_POINT('Origin',(-0.5111111111,0.,0.));
#52574=CARTESIAN_POINT('',(-1.,2.1388888889,19.3823413013222));
#52575=CARTESIAN_POINT('Origin',(-0.5111111111,0.4888888889,0.));
#52576=CARTESIAN_POINT('',(-0.5111111111,2.1388888889,0.));
#52577=CARTESIAN_POINT('',(-0.5111111111,-1.1611111111,0.));
#52578=CARTESIAN_POINT('Origin',(-1.,2.1388888889,0.));
#52579=CARTESIAN_POINT('',(-1.4888888889,2.1388888889,0.));
#52580=CARTESIAN_POINT('Origin',(0.00833333334999997,-1.1611111111,0.));
#52581=CARTESIAN_POINT('',(0.5277777778,-1.1611111111,0.));
#52582=CARTESIAN_POINT('Origin',(0.5277777778,-1.65,0.));
#52583=CARTESIAN_POINT('',(0.5277777778,-2.1388888889,0.));
#52584=CARTESIAN_POINT('Origin',(-1.,-2.1388888889,0.));
#52585=CARTESIAN_POINT('',(-2.5277777778,-2.1388888889,0.));
#52586=CARTESIAN_POINT('Origin',(-2.5277777778,-1.65,0.));
#52587=CARTESIAN_POINT('',(-2.5277777778,-1.1611111111,0.));
#52588=CARTESIAN_POINT('Origin',(-2.00833333335,-1.1611111111,0.));
#52589=CARTESIAN_POINT('',(-1.4888888889,-1.1611111111,0.));
#52590=CARTESIAN_POINT('Origin',(-1.4888888889,0.4888888889,0.));
#52591=CARTESIAN_POINT('Origin',(2.24242807365,1.24310434335,0.));
#52592=CARTESIAN_POINT('',(1.6994942043,2.1388888889,19.3823413013222));
#52593=CARTESIAN_POINT('',(1.6994942043,2.1388888889,0.));
#52594=CARTESIAN_POINT('',(2.785361943,0.3473197978,19.4969066510064));
#52595=CARTESIAN_POINT('Origin',(2.99587202900024,0.,0.));
#52596=CARTESIAN_POINT('',(2.785361943,0.3473197978,0.));
#52597=CARTESIAN_POINT('Origin',(1.127816949,2.1388888889,0.));
#52598=CARTESIAN_POINT('',(0.5561396937,2.1388888889,19.3823413013222));
#52599=CARTESIAN_POINT('',(0.5561396937,2.1388888889,0.));
#52600=CARTESIAN_POINT('',(1.127816949,2.1388888889,19.3823413013222));
#52601=CARTESIAN_POINT('Origin',(1.26544356065,0.9686111111,0.));
#52602=CARTESIAN_POINT('',(1.9747474276,-0.2016666667,19.4989571658472));
#52603=CARTESIAN_POINT('',(1.9747474276,-0.2016666667,0.));
#52604=CARTESIAN_POINT('Origin',(1.85251751839491,0.,0.));
#52605=CARTESIAN_POINT('Origin',(1.2577810923,-2.1388888889,0.));
#52606=CARTESIAN_POINT('',(1.8474876449,-2.1388888889,19.3823413013222));
#52607=CARTESIAN_POINT('',(1.8474876449,-2.1388888889,0.));
#52608=CARTESIAN_POINT('',(0.6680745397,-2.1388888889,19.3823413013222));
#52609=CARTESIAN_POINT('',(1.2577810923,-2.1388888889,19.3823413013222));
#52610=CARTESIAN_POINT('',(0.6680745397,-2.1388888889,0.));
#52611=CARTESIAN_POINT('Origin',(2.31642479395,-1.44366097505,0.));
#52612=CARTESIAN_POINT('',(2.785361943,-0.7484330612,19.4856318335563));
#52613=CARTESIAN_POINT('',(2.785361943,-0.7484330612,0.));
#52614=CARTESIAN_POINT('Origin',(3.29018641707832,0.,0.));
#52615=CARTESIAN_POINT('Origin',(2.785361943,-1.44366097505,0.));
#52616=CARTESIAN_POINT('',(2.785361943,-2.1388888889,19.3823413013222));
#52617=CARTESIAN_POINT('',(2.785361943,-2.1388888889,0.));
#52618=CARTESIAN_POINT('Origin',(2.785361943,0.,0.));
#52619=CARTESIAN_POINT('Origin',(3.2742508319,-2.1388888889,0.));
#52620=CARTESIAN_POINT('',(3.7631397208,-2.1388888889,19.3823413013222));
#52621=CARTESIAN_POINT('',(3.7631397208,-2.1388888889,0.));
#52622=CARTESIAN_POINT('',(3.2742508319,-2.1388888889,19.3823413013222));
#52623=CARTESIAN_POINT('Origin',(3.7631397208,0.,0.));
#52624=CARTESIAN_POINT('',(3.7631397208,2.1388888889,19.3823413013222));
#52625=CARTESIAN_POINT('',(3.7631397208,2.1388888889,0.));
#52626=CARTESIAN_POINT('Origin',(3.7631397208,0.,0.));
#52627=CARTESIAN_POINT('Origin',(3.2742508319,2.1388888889,0.));
#52628=CARTESIAN_POINT('',(2.785361943,2.1388888889,19.3823413013222));
#52629=CARTESIAN_POINT('',(2.785361943,2.1388888889,0.));
#52630=CARTESIAN_POINT('',(3.2742508319,2.1388888889,19.3823413013222));
#52631=CARTESIAN_POINT('Origin',(2.785361943,1.24310434335,0.));
#52632=CARTESIAN_POINT('Origin',(2.785361943,0.,0.));
#52633=CARTESIAN_POINT('Origin',(1.32141098365,-1.1702777778,0.));
#52634=CARTESIAN_POINT('Origin',(2.11077331185338,0.,0.));
#52635=CARTESIAN_POINT('Origin',(-1.,0.,0.));
#52636=CARTESIAN_POINT('Origin',(-1.,0.,0.));
#52637=CARTESIAN_POINT('',(-1.,5.5,18.7082869338697));
#52638=CARTESIAN_POINT('',(-5.7631397208,2.75,19.305115902268));
#52639=CARTESIAN_POINT('Origin',(-10.5262794424987,-5.18419751571741E-10,
-2.36643593609642E-9));
#52640=CARTESIAN_POINT('',(-3.8075841652,2.75,19.305115902268));
#52641=CARTESIAN_POINT('',(-4.785361943,2.75,19.305115902268));
#52642=CARTESIAN_POINT('',(-1.,4.3709594736,19.0038078626402));
#52643=CARTESIAN_POINT('Origin',(-8.570723907158,-1.22962007242933E-8,-6.41915343102539E-8));
#52644=CARTESIAN_POINT('',(1.8075841652,2.75,19.305115902268));
#52645=CARTESIAN_POINT('Origin',(6.57072388594774,-4.93771690202038E-11,
-4.65181226871891E-10));
#52646=CARTESIAN_POINT('',(3.7631397208,2.75,19.305115902268));
#52647=CARTESIAN_POINT('',(2.785361943,2.75,19.305115902268));
#52648=CARTESIAN_POINT('Origin',(8.5262794404497,6.64190369370488E-10,3.11044967560292E-9));
#52649=CARTESIAN_POINT('Origin',(-2.4037920826,3.5604797368,0.));
#52650=CARTESIAN_POINT('',(-1.,4.3709594736,0.));
#52651=CARTESIAN_POINT('',(-3.8075841652,2.75,0.));
#52652=CARTESIAN_POINT('Origin',(0.4037920826,3.5604797368,0.));
#52653=CARTESIAN_POINT('',(1.8075841652,2.75,0.));
#52654=CARTESIAN_POINT('Origin',(-4.785361943,2.75,0.));
#52655=CARTESIAN_POINT('',(-5.7631397208,2.75,0.));
#52656=CARTESIAN_POINT('Origin',(-3.3815698604,4.125,0.));
#52657=CARTESIAN_POINT('',(-1.,5.5,0.));
#52658=CARTESIAN_POINT('Origin',(1.3815698604,4.125,0.));
#52659=CARTESIAN_POINT('',(3.7631397208,2.75,0.));
#52660=CARTESIAN_POINT('Origin',(2.785361943,2.75,0.));
#52661=CARTESIAN_POINT('Origin',(-4.785361943,-2.75,0.));
#52662=CARTESIAN_POINT('',(-5.7631397208,-2.75,19.305115902268));
#52663=CARTESIAN_POINT('',(-5.7631397208,-2.75,0.));
#52664=CARTESIAN_POINT('',(-3.8075841652,-2.75,19.305115902268));
#52665=CARTESIAN_POINT('',(-4.785361943,-2.75,19.305115902268));
#52666=CARTESIAN_POINT('',(-3.8075841652,-2.75,0.));
#52667=CARTESIAN_POINT('Origin',(-3.3815698604,-4.125,0.));
#52668=CARTESIAN_POINT('',(-1.,-5.5,18.7082869338697));
#52669=CARTESIAN_POINT('',(-1.,-5.5,0.));
#52670=CARTESIAN_POINT('Origin',(-10.5262794400813,-8.77110606367637E-10,
4.09533296164E-9));
#52671=CARTESIAN_POINT('Origin',(1.3815698604,-4.125,0.));
#52672=CARTESIAN_POINT('',(3.7631397208,-2.75,19.305115902268));
#52673=CARTESIAN_POINT('',(3.7631397208,-2.75,0.));
#52674=CARTESIAN_POINT('Origin',(8.52627944078166,-4.73031613879016E-10,
2.23582041769532E-9));
#52675=CARTESIAN_POINT('Origin',(2.785361943,-2.75,0.));
#52676=CARTESIAN_POINT('',(1.8075841652,-2.75,19.305115902268));
#52677=CARTESIAN_POINT('',(1.8075841652,-2.75,0.));
#52678=CARTESIAN_POINT('',(2.785361943,-2.75,19.305115902268));
#52679=CARTESIAN_POINT('Origin',(-2.4037920826,-3.5604797368,0.));
#52680=CARTESIAN_POINT('',(-1.,-4.3709594736,19.0038078626402));
#52681=CARTESIAN_POINT('Origin',(-8.57072389406941,4.73950212409591E-9,
-2.49748000058503E-8));
#52682=CARTESIAN_POINT('',(-1.,-4.3709594736,0.));
#52683=CARTESIAN_POINT('Origin',(0.4037920826,-3.5604797368,0.));
#52684=CARTESIAN_POINT('Origin',(6.57072389929174,7.75191022484023E-9,-4.058589020417E-8));
#52685=CARTESIAN_POINT('Origin',(-1.,0.,0.));
#52686=CARTESIAN_POINT('Origin',(-4.4794070911,1.4086111111,0.));
#52687=CARTESIAN_POINT('',(-4.7295794663,2.1388888889,19.3823413013222));
#52688=CARTESIAN_POINT('',(-4.7295794663,2.1388888889,0.));
#52689=CARTESIAN_POINT('',(-4.2292347159,0.6783333333,19.4881980667514));
#52690=CARTESIAN_POINT('Origin',(-3.99710417002144,0.000721430429313635,
-2.2697089266716));
#52691=CARTESIAN_POINT('',(-4.2292347159,0.6783333333,0.));
#52692=CARTESIAN_POINT('Origin',(-5.24635959355,2.1388888889,0.));
#52693=CARTESIAN_POINT('',(-5.7631397208,2.1388888889,19.3823413013222));
#52694=CARTESIAN_POINT('',(-5.7631397208,2.1388888889,0.));
#52695=CARTESIAN_POINT('',(-5.24635959355,2.1388888889,19.3823413013222));
#52696=CARTESIAN_POINT('Origin',(-5.47540903359635,1.29897470288934,0.));
#52697=CARTESIAN_POINT('',(-5.18767834635794,0.459060516890588,19.4945957496387));
#52698=CARTESIAN_POINT('',(-5.18767834635794,0.459060516890588,0.));
#52699=CARTESIAN_POINT('Origin',(-5.03060343765304,0.000543454432446466,
-2.27211957514992));
#52700=CARTESIAN_POINT('Origin',(-4.3435534146,-0.7027777778,0.));
#52701=CARTESIAN_POINT('',(-4.3435534146,-2.1388888889,19.3823413013222));
#52702=CARTESIAN_POINT('',(-4.3435534146,-2.1388888889,0.));
#52703=CARTESIAN_POINT('Ctrl Pts',(-4.3435534146,-2.1388888889,19.3823413013222));
#52704=CARTESIAN_POINT('Ctrl Pts',(-4.52395809426988,-2.1388888889,19.3823413013222));
#52705=CARTESIAN_POINT('Ctrl Pts',(-4.71629563622818,-2.10281731621556,
19.3864277949426));
#52706=CARTESIAN_POINT('Ctrl Pts',(-5.06994974058055,-1.95633107681449,
19.4017574464858));
#52707=CARTESIAN_POINT('Ctrl Pts',(-5.23127577915034,-1.84592395078976,
19.4128536921776));
#52708=CARTESIAN_POINT('Ctrl Pts',(-5.48621793448543,-1.59118019669263,
19.4353935671731));
#52709=CARTESIAN_POINT('Ctrl Pts',(-5.59680474635876,-1.42973736216137,
19.4483236475342));
#52710=CARTESIAN_POINT('Ctrl Pts',(-5.74353126970954,-1.07583427316188,
19.4711073706637));
#52711=CARTESIAN_POINT('Ctrl Pts',(-5.7796645257,-0.883362239425408,19.4808193953452));
#52712=CARTESIAN_POINT('Ctrl Pts',(-5.7796645257,-0.522566272387348,19.4938308937715));
#52713=CARTESIAN_POINT('Ctrl Pts',(-5.74366463353765,-0.330266483099083,
19.4980055699564));
#52714=CARTESIAN_POINT('Ctrl Pts',(-5.59716211486846,0.0235426180269262,
19.500788263579));
#52715=CARTESIAN_POINT('Ctrl Pts',(-5.48665892619763,0.185050560069143,
19.4995390181328));
#52716=CARTESIAN_POINT('Ctrl Pts',(-5.30716969365494,0.364587581151339,
19.4966607992451));
#52717=CARTESIAN_POINT('Ctrl Pts',(-5.24968384954062,0.414010881858001,
19.495656582549));
#52718=CARTESIAN_POINT('Ctrl Pts',(-5.18767834635794,0.459060516890588,
19.4945957496387));
#52719=CARTESIAN_POINT('Origin',(-3.54299785905,-2.1388888889,0.));
#52720=CARTESIAN_POINT('',(-2.7424423035,-2.1388888889,19.3823413013222));
#52721=CARTESIAN_POINT('',(-2.7424423035,-2.1388888889,0.));
#52722=CARTESIAN_POINT('',(-3.54299785905,-2.1388888889,19.3823413013222));
#52723=CARTESIAN_POINT('Origin',(-3.7202200813,-0.7027777778,0.));
#52724=CARTESIAN_POINT('',(-3.7202200813,-1.1061111111,19.468603396492));
#52725=CARTESIAN_POINT('',(-3.7202200813,-1.1061111111,0.));
#52726=CARTESIAN_POINT('',(-3.7202200813,-0.2994444445,19.497700711229));
#52727=CARTESIAN_POINT('Origin',(-3.7202200813,0.,0.));
#52728=CARTESIAN_POINT('',(-3.7202200813,-0.2994444445,0.));
#52729=CARTESIAN_POINT('Origin',(-4.03188674795,-1.1061111111,0.));
#52730=CARTESIAN_POINT('',(-4.3435534146,-1.1061111111,19.468603396492));
#52731=CARTESIAN_POINT('',(-4.3435534146,-1.1061111111,0.));
#52732=CARTESIAN_POINT('',(-4.03188674795,-1.1061111111,19.468603396492));
#52733=CARTESIAN_POINT('Origin',(-2.7424423035,0.,0.));
#52734=CARTESIAN_POINT('',(-2.7424423035,2.1388888889,19.3823413013222));
#52735=CARTESIAN_POINT('',(-2.7424423035,2.1388888889,0.));
#52736=CARTESIAN_POINT('Origin',(-2.7424423035,0.,0.));
#52737=CARTESIAN_POINT('Origin',(-3.2313311924,2.1388888889,0.));
#52738=CARTESIAN_POINT('',(-3.7202200813,2.1388888889,19.3823413013222));
#52739=CARTESIAN_POINT('',(-3.7202200813,2.1388888889,0.));
#52740=CARTESIAN_POINT('',(-3.2313311924,2.1388888889,19.3823413013222));
#52741=CARTESIAN_POINT('Origin',(-3.7202200813,1.4086111111,0.));
#52742=CARTESIAN_POINT('',(-3.7202200813,0.6783333333,19.4881980667514));
#52743=CARTESIAN_POINT('',(-3.7202200813,0.6783333333,0.));
#52744=CARTESIAN_POINT('Origin',(-3.7202200813,0.,0.));
#52745=CARTESIAN_POINT('Origin',(-3.9747273986,0.6783333333,0.));
#52746=CARTESIAN_POINT('',(-3.9747273986,0.6783333333,19.4881980667514));
#52747=CARTESIAN_POINT('Origin',(-4.3435534146,-0.7027777778,0.));
#52748=CARTESIAN_POINT('',(-4.3435534146,-0.2994444445,19.497700711229));
#52749=CARTESIAN_POINT('',(-4.3435534146,-0.2994444445,0.));
#52750=CARTESIAN_POINT('Ctrl Pts',(-4.3435534146,-1.1061111111,19.468603396492));
#52751=CARTESIAN_POINT('Ctrl Pts',(-4.39419814308983,-1.1061111111,19.468603396492));
#52752=CARTESIAN_POINT('Ctrl Pts',(-4.44821225425436,-1.0959892259289,19.4691867368818));
#52753=CARTESIAN_POINT('Ctrl Pts',(-4.54756315899303,-1.0548413233652,19.4714594820528));
#52754=CARTESIAN_POINT('Ctrl Pts',(-4.59290043242865,-1.02381583731486,
19.4731375157807));
#52755=CARTESIAN_POINT('Ctrl Pts',(-4.66452631029908,-0.952218736036693,
19.4767698957415));
#52756=CARTESIAN_POINT('Ctrl Pts',(-4.69557900256288,-0.906859343552727,
19.4789650772337));
#52757=CARTESIAN_POINT('Ctrl Pts',(-4.73675930343402,-0.807469845951887,
19.4833381841241));
#52758=CARTESIAN_POINT('Ctrl Pts',(-4.7468867479,-0.75343917779947,19.4855048515763));
#52759=CARTESIAN_POINT('Ctrl Pts',(-4.7468867479,-0.652145736281435,19.4891578288136));
#52760=CARTESIAN_POINT('Ctrl Pts',(-4.73676979677675,-0.598128620436881,
19.4908879558739));
#52761=CARTESIAN_POINT('Ctrl Pts',(-4.69560712746241,-0.498746523663012,
19.4936841838618));
#52762=CARTESIAN_POINT('Ctrl Pts',(-4.66456102115108,-0.453382021110974,
19.4947615621894));
#52763=CARTESIAN_POINT('Ctrl Pts',(-4.59293064696051,-0.381759433086016,
19.4962956016238));
#52764=CARTESIAN_POINT('Ctrl Pts',(-4.54757997199792,-0.350722506379112,
19.4968566012566));
#52765=CARTESIAN_POINT('Ctrl Pts',(-4.44821221942384,-0.309565004720403,
19.4975535161267));
#52766=CARTESIAN_POINT('Ctrl Pts',(-4.39419521514208,-0.2994444445,19.497700711229));
#52767=CARTESIAN_POINT('Ctrl Pts',(-4.3435534146,-0.2994444445,19.497700711229));
#52768=CARTESIAN_POINT('Origin',(-4.03188674795,-0.2994444445,0.));
#52769=CARTESIAN_POINT('',(-4.03188674795,-0.2994444445,19.497700711229));
#52770=CARTESIAN_POINT('Origin',(-1.,0.,0.));
#57024=UNCERTAINTY_MEASURE_WITH_UNIT(LENGTH_MEASURE(0.01),#57080,
'DISTANCE_ACCURACY_VALUE',
'Maximum model space distance between geometric entities at asserted c
onnectivities');
#57040=UNCERTAINTY_MEASURE_WITH_UNIT(LENGTH_MEASURE(0.01),#57080,
'DISTANCE_ACCURACY_VALUE',
'Maximum model space distance between geometric entities at asserted c
onnectivities');
#57063=(
GEOMETRIC_REPRESENTATION_CONTEXT(3)
GLOBAL_UNCERTAINTY_ASSIGNED_CONTEXT((#57024))
GLOBAL_UNIT_ASSIGNED_CONTEXT((#57080,#57082,#57083))
REPRESENTATION_CONTEXT('','3D')
);
#57079=(
GEOMETRIC_REPRESENTATION_CONTEXT(3)
GLOBAL_UNCERTAINTY_ASSIGNED_CONTEXT((#57040))
GLOBAL_UNIT_ASSIGNED_CONTEXT((#57080,#57082,#57083))
REPRESENTATION_CONTEXT('','3D')
);
#57080=(
LENGTH_UNIT()
NAMED_UNIT(*)
SI_UNIT(.MILLI.,.METRE.)
);
#57082=(
NAMED_UNIT(*)
PLANE_ANGLE_UNIT()
SI_UNIT($,.RADIAN.)
);
#57083=(
NAMED_UNIT(*)
SI_UNIT($,.STERADIAN.)
SOLID_ANGLE_UNIT()
);
#57106=SHAPE_DEFINITION_REPRESENTATION(#57152,#57271);
#57152=PRODUCT_DEFINITION_SHAPE('',$,#57310);
#57271=SHAPE_REPRESENTATION('',(#25820),#57063);
#57287=PRODUCT_DEFINITION_CONTEXT('part definition',#57403,'design');
#57310=PRODUCT_DEFINITION('Coupling Hub 2','Coupling Hub 2',#57348,#57287);
#57348=PRODUCT_DEFINITION_FORMATION('',$,#57427);
#57403=APPLICATION_CONTEXT(
'Core Data for Automotive Mechanical Design Process');
#57404=PRODUCT_CONTEXT('part definition',#57403,'mechanical');
#57427=PRODUCT('Coupling Hub 2','Coupling Hub 2',$,(#57404));
#57444=PRESENTATION_STYLE_ASSIGNMENT((#57446));
#57446=SURFACE_STYLE_USAGE(.BOTH.,#57448);
#57448=SURFACE_SIDE_STYLE('',(#57450));
#57450=SURFACE_STYLE_FILL_AREA(#57452);
#57452=FILL_AREA_STYLE('Opaque(202,209,238)',(#57454));
#57454=FILL_AREA_STYLE_COLOUR('Opaque(202,209,238)',#57456);
#57456=COLOUR_RGB('Opaque(202,209,238)',0.792156862745098,0.819607843137255,
0.933333333333333);
ENDSEC;
END-ISO-10303-21;
